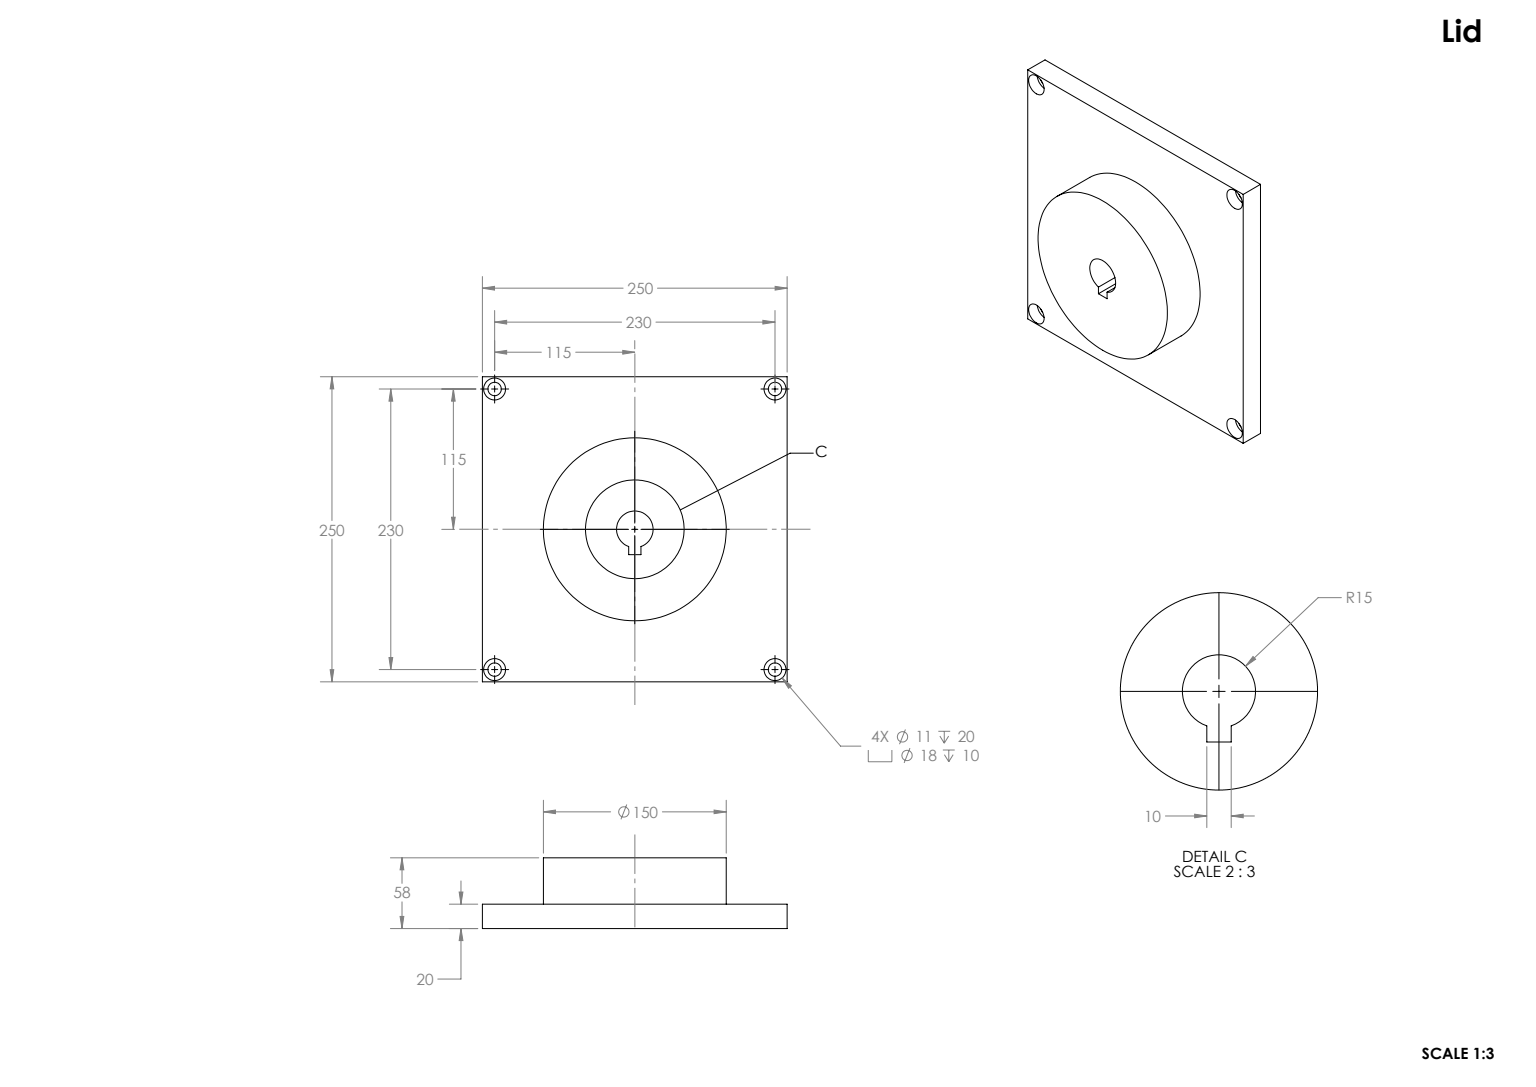
ISO-10303-21;
HEADER;
FILE_DESCRIPTION (('STEP AP214'),
    '1' );
FILE_NAME ('Lid.step',
    '2026-10-28T15:55:38',
    ( '' ),
    ( '' ),
    'SwSTEP 2.0',
    'SolidWorks 2025',
    '' );
FILE_SCHEMA (( 'AUTOMOTIVE_DESIGN' ));
ENDSEC;

DATA;
#6=AXIS2_PLACEMENT_3D ( 'NONE', #6964, #1191, #3754 ) ;
#14=VERTEX_POINT ( 'NONE', #1674 ) ;
#22=DIRECTION ( 'NONE',  ( -0.000000000000000000, -0.000000000000000000, 1.000000000000000000 ) ) ;
#33=ADVANCED_FACE ( 'NONE', ( #7283, #3451 ), #1624, .F. ) ;
#45=CARTESIAN_POINT ( 'NONE',  ( 0.000000000000000000, 0.000000000000000000, 57.99999999999999289 ) ) ;
#51=EDGE_CURVE ( 'NONE', #2241, #1087, #5313, .T. ) ;
#54=CARTESIAN_POINT ( 'NONE',  ( 115.0000000000000000, 114.9999999999999716, 10.00000000000000000 ) ) ;
#57=VERTEX_POINT ( 'NONE', #5409 ) ;
#69=VECTOR ( 'NONE', #3861, 1000.000000000000000 ) ;
#73=DIRECTION ( 'NONE',  ( -1.000000000000000000, -0.000000000000000000, -0.000000000000000000 ) ) ;
#77=APPLICATION_CONTEXT ( 'automotive_design' ) ;
#85=ORIENTED_EDGE ( 'NONE', *, *, #3477, .F. ) ;
#88=AXIS2_PLACEMENT_3D ( 'NONE', #5932, #1987, #3343 ) ;
#95=DIRECTION ( 'NONE',  ( -0.000000000000000000, -0.000000000000000000, 1.000000000000000000 ) ) ;
#99=ORIENTED_EDGE ( 'NONE', *, *, #619, .T. ) ;
#103=FACE_OUTER_BOUND ( 'NONE', #252, .T. ) ;
#107=CIRCLE ( 'NONE', #1347, 5.499999999999991118 ) ;
#117=FACE_OUTER_BOUND ( 'NONE', #1113, .T. ) ;
#119=AXIS2_PLACEMENT_3D ( 'NONE', #3115, #5695, #7738 ) ;
#121=DIRECTION ( 'NONE',  ( -0.000000000000000000, -0.000000000000000000, 1.000000000000000000 ) ) ;
#125=ORIENTED_EDGE ( 'NONE', *, *, #5217, .T. ) ;
#126=PLANE ( 'NONE',  #6282 ) ;
#129=ORIENTED_EDGE ( 'NONE', *, *, #3717, .T. ) ;
#133=CARTESIAN_POINT ( 'NONE',  ( 14.14213562373095279, -5.000000000000000000, 0.000000000000000000 ) ) ;
#134=ADVANCED_FACE ( 'NONE', ( #2899 ), #7943, .F. ) ;
#140=AXIS2_PLACEMENT_3D ( 'NONE', #6010, #7299, #1005 ) ;
#144=CARTESIAN_POINT ( 'NONE',  ( -109.5000000000000000, -114.9999999999999858, 20.00000000000000000 ) ) ;
#153=VERTEX_POINT ( 'NONE', #5449 ) ;
#156=DIRECTION ( 'NONE',  ( 1.000000000000000000, 0.000000000000000000, 0.000000000000000000 ) ) ;
#166=CARTESIAN_POINT ( 'NONE',  ( 124.9999999999997442, -125.0000000000000000, 20.00000000000000000 ) ) ;
#189=EDGE_CURVE ( 'NONE', #2853, #6262, #8132, .T. ) ;
#197=CARTESIAN_POINT ( 'NONE',  ( 115.0000000000000000, 114.9999999999999716, 10.00000000000000000 ) ) ;
#218=ORIENTED_EDGE ( 'NONE', *, *, #2588, .F. ) ;
#235=DIRECTION ( 'NONE',  ( 1.000000000000000000, 0.000000000000000000, 0.000000000000000000 ) ) ;
#252=EDGE_LOOP ( 'NONE', ( #5794, #5594, #8327, #2636 ) ) ;
#253=VECTOR ( 'NONE', #4816, 1000.000000000000000 ) ;
#258=ADVANCED_FACE ( 'NONE', ( #117 ), #4551, .F. ) ;
#259=DIRECTION ( 'NONE',  ( 9.992007221626408864E-16, 1.000000000000000000, 0.000000000000000000 ) ) ;
#268=VERTEX_POINT ( 'NONE', #3361 ) ;
#273=ORIENTED_EDGE ( 'NONE', *, *, #5206, .F. ) ;
#274=DIRECTION ( 'NONE',  ( 0.000000000000000000, -0.000000000000000000, -1.000000000000000000 ) ) ;
#283=ADVANCED_FACE ( 'NONE', ( #3284, #3966, #689, #5244, #1367, #6459 ), #5952, .F. ) ;
#284=EDGE_CURVE ( 'NONE', #5879, #3698, #7868, .T. ) ;
#290=ORIENTED_EDGE ( 'NONE', *, *, #7886, .F. ) ;
#293=VERTEX_POINT ( 'NONE', #814 ) ;
#299=APPLICATION_CONTEXT ( 'automotive_design' ) ;
#312=EDGE_LOOP ( 'NONE', ( #3163, #5141 ) ) ;
#317=CARTESIAN_POINT ( 'NONE',  ( 125.0000000000000000, 125.0000000000000000, 0.000000000000000000 ) ) ;
#322=DIRECTION ( 'NONE',  ( -0.000000000000000000, -0.000000000000000000, -1.000000000000000000 ) ) ;
#351=VERTEX_POINT ( 'NONE', #1784 ) ;
#353=DIRECTION ( 'NONE',  ( 1.000000000000000000, 0.000000000000000000, 0.000000000000000000 ) ) ;
#361=DIRECTION ( 'NONE',  ( 1.000000000000000000, 0.000000000000000000, 0.000000000000000000 ) ) ;
#365=ORIENTED_EDGE ( 'NONE', *, *, #7229, .F. ) ;
#369=CARTESIAN_POINT ( 'NONE',  ( 20.76917701662883076, -5.000000000000000000, 0.000000000000000000 ) ) ;
#372=VERTEX_POINT ( 'NONE', #4240 ) ;
#379=ORIENTED_EDGE ( 'NONE', *, *, #688, .F. ) ;
#426=VERTEX_POINT ( 'NONE', #6449 ) ;
#432=CARTESIAN_POINT ( 'NONE',  ( 124.0000000000000000, 114.9999999999999716, 10.00000000000000000 ) ) ;
#438=ORIENTED_EDGE ( 'NONE', *, *, #5217, .F. ) ;
#442=LINE ( 'NONE', #6912, #6022 ) ;
#449=DIRECTION ( 'NONE',  ( -1.000000000000000000, 0.000000000000000000, -0.000000000000000000 ) ) ;
#462=EDGE_CURVE ( 'NONE', #1143, #501, #4654, .T. ) ;
#464=( GEOMETRIC_REPRESENTATION_CONTEXT ( 3 ) GLOBAL_UNCERTAINTY_ASSIGNED_CONTEXT ( ( #4359 ) ) GLOBAL_UNIT_ASSIGNED_CONTEXT ( ( #3691, #7766, #3944 ) ) REPRESENTATION_CONTEXT ( 'NONE', 'WORKASPACE' ) );
#482=CIRCLE ( 'NONE', #7640, 8.999999999999994671 ) ;
#498=DIRECTION ( 'NONE',  ( -1.000000000000000000, -0.000000000000000000, -0.000000000000000000 ) ) ;
#501=VERTEX_POINT ( 'NONE', #1652 ) ;
#504=AXIS2_PLACEMENT_3D ( 'NONE', #7381, #3470, #967 ) ;
#514=ORIENTED_EDGE ( 'NONE', *, *, #1744, .T. ) ;
#521=ORIENTED_EDGE ( 'NONE', *, *, #5929, .F. ) ;
#542=ORIENTED_EDGE ( 'NONE', *, *, #6069, .T. ) ;
#561=EDGE_LOOP ( 'NONE', ( #1225, #8285, #5177, #3711 ) ) ;
#571=EDGE_LOOP ( 'NONE', ( #8103, #3538 ) ) ;
#572=CARTESIAN_POINT ( 'NONE',  ( 0.000000000000000000, 0.000000000000000000, 57.99999999999999289 ) ) ;
#574=CARTESIAN_POINT ( 'NONE',  ( -105.9999999999999858, -114.9999999999999858, 20.00000000000000000 ) ) ;
#577=AXIS2_PLACEMENT_3D ( 'NONE', #4578, #1221, #3947 ) ;
#586=LINE ( 'NONE', #6396, #3892 ) ;
#601=ORIENTED_EDGE ( 'NONE', *, *, #7179, .F. ) ;
#616=DIRECTION ( 'NONE',  ( -0.000000000000000000, -0.000000000000000000, 1.000000000000000000 ) ) ;
#619=EDGE_CURVE ( 'NONE', #372, #3698, #5183, .T. ) ;
#625=EDGE_LOOP ( 'NONE', ( #5499, #7571, #8014, #125 ) ) ;
#627=AXIS2_PLACEMENT_3D ( 'NONE', #6959, #2577, #1183 ) ;
#634=ORIENTED_EDGE ( 'NONE', *, *, #7886, .T. ) ;
#653=VERTEX_POINT ( 'NONE', #4478 ) ;
#655=CYLINDRICAL_SURFACE ( 'NONE', #1454, 75.00000000000001421 ) ;
#664=EDGE_CURVE ( 'NONE', #8205, #351, #3409, .T. ) ;
#667=ORIENTED_EDGE ( 'NONE', *, *, #3851, .F. ) ;
#669=CARTESIAN_POINT ( 'NONE',  ( 120.5000000000000000, 114.9999999999999716, 10.00000000000000000 ) ) ;
#685=VECTOR ( 'NONE', #498, 1000.000000000000000 ) ;
#686=CARTESIAN_POINT ( 'NONE',  ( -120.4999999999999858, -114.9999999999999858, 0.000000000000000000 ) ) ;
#688=EDGE_CURVE ( 'NONE', #7860, #57, #8154, .T. ) ;
#689=FACE_BOUND ( 'NONE', #7167, .T. ) ;
#716=CARTESIAN_POINT ( 'NONE',  ( 106.0000000000000142, -114.9999999999999716, 20.00000000000000000 ) ) ;
#719=VECTOR ( 'NONE', #8002, 1000.000000000000000 ) ;
#725=ADVANCED_FACE ( 'NONE', ( #4875 ), #7426, .F. ) ;
#732=LINE ( 'NONE', #8263, #8074 ) ;
#758=VERTEX_POINT ( 'NONE', #317 ) ;
#759=DIRECTION ( 'NONE',  ( -0.000000000000000000, -0.000000000000000000, 1.000000000000000000 ) ) ;
#768=DIRECTION ( 'NONE',  ( 1.000000000000000000, 0.000000000000000000, 0.000000000000000000 ) ) ;
#771=CARTESIAN_POINT ( 'NONE',  ( 75.00000000000001421, 9.184850993605150311E-15, 57.99999999999999289 ) ) ;
#780=CIRCLE ( 'NONE', #5493, 5.499999999999991118 ) ;
#790=VECTOR ( 'NONE', #7088, 1000.000000000000000 ) ;
#794=DIRECTION ( 'NONE',  ( -0.000000000000000000, -0.000000000000000000, 1.000000000000000000 ) ) ;
#799=AXIS2_PLACEMENT_3D ( 'NONE', #2892, #1645, #6922 ) ;
#809=ORIENTED_EDGE ( 'NONE', *, *, #1189, .T. ) ;
#814=CARTESIAN_POINT ( 'NONE',  ( 106.0000000000000142, 114.9999999999999716, 20.00000000000000000 ) ) ;
#818=DIRECTION ( 'NONE',  ( 1.000000000000000000, -9.992007221626408864E-16, 0.000000000000000000 ) ) ;
#826=MANIFOLD_SOLID_BREP ( 'CBORE for M10 SHCS1', #2352 ) ;
#837=EDGE_LOOP ( 'NONE', ( #1271, #3506, #2194, #809 ) ) ;
#844=CARTESIAN_POINT ( 'NONE',  ( -114.9999999999999716, 114.9999999999999858, 0.000000000000000000 ) ) ;
#853=CARTESIAN_POINT ( 'NONE',  ( 115.0000000000000000, -114.9999999999999716, 10.00000000000000000 ) ) ;
#873=AXIS2_PLACEMENT_3D ( 'NONE', #2320, #8006, #5392 ) ;
#886=DIRECTION ( 'NONE',  ( -0.000000000000000000, -0.000000000000000000, 1.000000000000000000 ) ) ;
#891=ADVANCED_BREP_SHAPE_REPRESENTATION ( '', ( #826, #1299 ), #3387 ) ;
#893=FACE_BOUND ( 'NONE', #1076, .T. ) ;
#898=LINE ( 'NONE', #5411, #1902 ) ;
#905=CARTESIAN_POINT ( 'NONE',  ( 0.000000000000000000, -5.000000000000000000, 57.99999999999999289 ) ) ;
#919=DIRECTION ( 'NONE',  ( -0.000000000000000000, -0.000000000000000000, 1.000000000000000000 ) ) ;
#924=ORIENTED_EDGE ( 'NONE', *, *, #2528, .T. ) ;
#927=AXIS2_PLACEMENT_3D ( 'NONE', #5655, #7690, #1908 ) ;
#929=VERTEX_POINT ( 'NONE', #6649 ) ;
#964=CARTESIAN_POINT ( 'NONE',  ( 115.0000000000000000, -114.9999999999999716, 0.000000000000000000 ) ) ;
#967=DIRECTION ( 'NONE',  ( 1.000000000000000000, 0.000000000000000000, 0.000000000000000000 ) ) ;
#971=FACE_OUTER_BOUND ( 'NONE', #1682, .T. ) ;
#979=DIRECTION ( 'NONE',  ( 1.000000000000000000, 0.000000000000000000, 0.000000000000000000 ) ) ;
#989=DIRECTION ( 'NONE',  ( -1.000000000000000000, 0.000000000000000000, -0.000000000000000000 ) ) ;
#992=CARTESIAN_POINT ( 'NONE',  ( -124.0000000000000000, -114.9999999999999858, 20.00000000000000000 ) ) ;
#995=LINE ( 'NONE', #2149, #5893 ) ;
#1005=DIRECTION ( 'NONE',  ( 1.000000000000000000, 0.000000000000000000, 0.000000000000000000 ) ) ;
#1009=DIRECTION ( 'NONE',  ( -0.000000000000000000, -0.000000000000000000, 1.000000000000000000 ) ) ;
#1014=DIRECTION ( 'NONE',  ( -9.992007221626408864E-16, -1.000000000000000000, -0.000000000000000000 ) ) ;
#1041=ORIENTED_EDGE ( 'NONE', *, *, #7075, .T. ) ;
#1047=AXIS2_PLACEMENT_3D ( 'NONE', #6210, #2387, #6762 ) ;
#1053=CARTESIAN_POINT ( 'NONE',  ( -125.0000000000000000, 125.0000000000000000, 20.00000000000000000 ) ) ;
#1065=CIRCLE ( 'NONE', #799, 8.999999999999994671 ) ;
#1076=EDGE_LOOP ( 'NONE', ( #5400, #6032 ) ) ;
#1078=( NAMED_UNIT ( * ) PLANE_ANGLE_UNIT ( ) SI_UNIT ( $, .RADIAN. ) );
#1087=VERTEX_POINT ( 'NONE', #3806 ) ;
#1089=EDGE_CURVE ( 'NONE', #6262, #268, #5748, .T. ) ;
#1105=ORIENTED_EDGE ( 'NONE', *, *, #2915, .T. ) ;
#1113=EDGE_LOOP ( 'NONE', ( #6418, #4791, #1621, #1265 ) ) ;
#1121=CARTESIAN_POINT ( 'NONE',  ( -125.0000000000002558, -125.0000000000000000, 0.000000000000000000 ) ) ;
#1131=DIRECTION ( 'NONE',  ( 0.000000000000000000, 0.000000000000000000, 1.000000000000000000 ) ) ;
#1143=VERTEX_POINT ( 'NONE', #686 ) ;
#1145=ORIENTED_EDGE ( 'NONE', *, *, #664, .F. ) ;
#1158=CARTESIAN_POINT ( 'NONE',  ( 115.0000000000000000, 114.9999999999999716, 0.000000000000000000 ) ) ;
#1165=EDGE_LOOP ( 'NONE', ( #6743, #6397, #4823, #4757 ) ) ;
#1172=LINE ( 'NONE', #2644, #69 ) ;
#1175=ORIENTED_EDGE ( 'NONE', *, *, #6340, .F. ) ;
#1183=DIRECTION ( 'NONE',  ( 1.000000000000000000, 0.000000000000000000, 0.000000000000000000 ) ) ;
#1187=PRODUCT_CONTEXT ( 'NONE', #77, 'mechanical' ) ;
#1189=EDGE_CURVE ( 'NONE', #5618, #268, #5155, .T. ) ;
#1191=DIRECTION ( 'NONE',  ( 0.000000000000000000, 0.000000000000000000, 1.000000000000000000 ) ) ;
#1192=VECTOR ( 'NONE', #2719, 1000.000000000000000 ) ;
#1199=VERTEX_POINT ( 'NONE', #2217 ) ;
#1200=CIRCLE ( 'NONE', #6849, 5.499999999999991118 ) ;
#1202=DIRECTION ( 'NONE',  ( 1.000000000000000000, 0.000000000000000000, 0.000000000000000000 ) ) ;
#1207=VERTEX_POINT ( 'NONE', #7349 ) ;
#1208=EDGE_CURVE ( 'NONE', #5352, #293, #1483, .T. ) ;
#1221=DIRECTION ( 'NONE',  ( -1.000000000000000000, 9.992007221626408864E-16, 0.000000000000000000 ) ) ;
#1225=ORIENTED_EDGE ( 'NONE', *, *, #1208, .F. ) ;
#1263=ORIENTED_EDGE ( 'NONE', *, *, #2767, .T. ) ;
#1265=ORIENTED_EDGE ( 'NONE', *, *, #1711, .T. ) ;
#1271=ORIENTED_EDGE ( 'NONE', *, *, #1089, .F. ) ;
#1294=VERTEX_POINT ( 'NONE', #5614 ) ;
#1296=CARTESIAN_POINT ( 'NONE',  ( -114.9999999999999858, -114.9999999999999858, 10.00000000000000000 ) ) ;
#1299=AXIS2_PLACEMENT_3D ( 'NONE', #5884, #1507, #5927 ) ;
#1300=ORIENTED_EDGE ( 'NONE', *, *, #2228, .F. ) ;
#1308=VECTOR ( 'NONE', #4861, 1000.000000000000000 ) ;
#1340=LINE ( 'NONE', #3907, #3449 ) ;
#1347=AXIS2_PLACEMENT_3D ( 'NONE', #2247, #2924, #1634 ) ;
#1349=EDGE_LOOP ( 'NONE', ( #1695, #7646 ) ) ;
#1358=LINE ( 'NONE', #6493, #7675 ) ;
#1362=ADVANCED_FACE ( 'NONE', ( #1991 ), #4621, .F. ) ;
#1366=ORIENTED_EDGE ( 'NONE', *, *, #7946, .F. ) ;
#1367=FACE_BOUND ( 'NONE', #3037, .T. ) ;
#1368=CARTESIAN_POINT ( 'NONE',  ( 124.0000000000000000, 114.9999999999999716, 20.00000000000000000 ) ) ;
#1372=ORIENTED_EDGE ( 'NONE', *, *, #2788, .F. ) ;
#1381=DIRECTION ( 'NONE',  ( -0.000000000000000000, -0.000000000000000000, 1.000000000000000000 ) ) ;
#1385=ORIENTED_EDGE ( 'NONE', *, *, #6069, .F. ) ;
#1417=AXIS2_PLACEMENT_3D ( 'NONE', #7031, #4519, #5124 ) ;
#1431=ORIENTED_EDGE ( 'NONE', *, *, #2734, .T. ) ;
#1435=VECTOR ( 'NONE', #259, 1000.000000000000000 ) ;
#1444=ORIENTED_EDGE ( 'NONE', *, *, #3717, .F. ) ;
#1447=DIRECTION ( 'NONE',  ( -0.000000000000000000, -0.000000000000000000, 1.000000000000000000 ) ) ;
#1450=EDGE_CURVE ( 'NONE', #6338, #1207, #1511, .T. ) ;
#1453=FACE_BOUND ( 'NONE', #6015, .T. ) ;
#1454=AXIS2_PLACEMENT_3D ( 'NONE', #572, #1894, #6985 ) ;
#1471=AXIS2_PLACEMENT_3D ( 'NONE', #3560, #7559, #361 ) ;
#1477=LINE ( 'NONE', #7862, #1605 ) ;
#1483=LINE ( 'NONE', #6755, #2989 ) ;
#1487=PRODUCT_DEFINITION_SHAPE ( 'NONE', 'NONE',  #1686 ) ;
#1495=FACE_BOUND ( 'NONE', #2408, .T. ) ;
#1503=CARTESIAN_POINT ( 'NONE',  ( -109.5000000000000000, -114.9999999999999858, 10.00000000000000000 ) ) ;
#1505=DIRECTION ( 'NONE',  ( -1.000000000000000000, 0.000000000000000000, -0.000000000000000000 ) ) ;
#1507=DIRECTION ( 'NONE',  ( 0.000000000000000000, 0.000000000000000000, 1.000000000000000000 ) ) ;
#1511=LINE ( 'NONE', #7201, #4061 ) ;
#1515=LINE ( 'NONE', #7334, #5232 ) ;
#1519=AXIS2_PLACEMENT_3D ( 'NONE', #197, #2821, #156 ) ;
#1533=EDGE_CURVE ( 'NONE', #1199, #153, #4022, .T. ) ;
#1535=FACE_OUTER_BOUND ( 'NONE', #3964, .T. ) ;
#1538=ORIENTED_EDGE ( 'NONE', *, *, #5058, .F. ) ;
#1548=ORIENTED_EDGE ( 'NONE', *, *, #3525, .T. ) ;
#1552=ORIENTED_EDGE ( 'NONE', *, *, #1450, .T. ) ;
#1557=DIRECTION ( 'NONE',  ( 1.000000000000000000, 0.000000000000000000, 0.000000000000000000 ) ) ;
#1566=VERTEX_POINT ( 'NONE', #6176 ) ;
#1567=CARTESIAN_POINT ( 'NONE',  ( 125.0000000000000000, 125.0000000000000000, 20.00000000000000000 ) ) ;
#1568=DIRECTION ( 'NONE',  ( -0.000000000000000000, -0.000000000000000000, 1.000000000000000000 ) ) ;
#1605=VECTOR ( 'NONE', #2094, 1000.000000000000000 ) ;
#1615=CARTESIAN_POINT ( 'NONE',  ( 120.5000000000000000, 114.9999999999999716, 20.00000000000000000 ) ) ;
#1620=CIRCLE ( 'NONE', #7960, 75.00000000000001421 ) ;
#1621=ORIENTED_EDGE ( 'NONE', *, *, #7009, .T. ) ;
#1624=PLANE ( 'NONE',  #2738 ) ;
#1633=ORIENTED_EDGE ( 'NONE', *, *, #3223, .T. ) ;
#1634=DIRECTION ( 'NONE',  ( 1.000000000000000000, 0.000000000000000000, 0.000000000000000000 ) ) ;
#1636=EDGE_CURVE ( 'NONE', #3543, #5352, #2216, .T. ) ;
#1644=ORIENTED_EDGE ( 'NONE', *, *, #5930, .T. ) ;
#1645=DIRECTION ( 'NONE',  ( -0.000000000000000000, -0.000000000000000000, 1.000000000000000000 ) ) ;
#1652=CARTESIAN_POINT ( 'NONE',  ( -120.4999999999999858, -114.9999999999999858, 10.00000000000000000 ) ) ;
#1662=VERTEX_POINT ( 'NONE', #5987 ) ;
#1673=DIRECTION ( 'NONE',  ( 1.000000000000000000, 0.000000000000000000, 0.000000000000000000 ) ) ;
#1674=CARTESIAN_POINT ( 'NONE',  ( 120.5000000000000000, -114.9999999999999716, 0.000000000000000000 ) ) ;
#1682=EDGE_LOOP ( 'NONE', ( #8203, #4102, #5975, #2895 ) ) ;
#1686=PRODUCT_DEFINITION ( 'UNKNOWN', '', #2343, #7430 ) ;
#1695=ORIENTED_EDGE ( 'NONE', *, *, #189, .T. ) ;
#1698=EDGE_CURVE ( 'NONE', #3530, #2214, #6790, .T. ) ;
#1700=ADVANCED_FACE ( 'NONE', ( #6744 ), #8096, .F. ) ;
#1703=CIRCLE ( 'NONE', #4107, 9.000000000000007105 ) ;
#1708=SHAPE_REPRESENTATION ( 'Lid', ( #1299 ), #3387 ) ;
#1711=EDGE_CURVE ( 'NONE', #929, #501, #3521, .T. ) ;
#1721=AXIS2_PLACEMENT_3D ( 'NONE', #7158, #95, #6475 ) ;
#1727=AXIS2_PLACEMENT_3D ( 'NONE', #4123, #7941, #7907 ) ;
#1740=CARTESIAN_POINT ( 'NONE',  ( -114.9999999999999716, 114.9999999999999858, 10.00000000000000000 ) ) ;
#1744=EDGE_CURVE ( 'NONE', #3799, #4692, #4066, .T. ) ;
#1750=VECTOR ( 'NONE', #7803, 1000.000000000000000 ) ;
#1754=EDGE_LOOP ( 'NONE', ( #5016, #1300, #6482, #2342 ) ) ;
#1762=ORIENTED_EDGE ( 'NONE', *, *, #2056, .T. ) ;
#1779=SHAPE_DEFINITION_REPRESENTATION ( #1487, #1708 ) ;
#1784=CARTESIAN_POINT ( 'NONE',  ( 14.14213562373095279, -5.000000000000000000, 0.000000000000000000 ) ) ;
#1791=ORIENTED_EDGE ( 'NONE', *, *, #1450, .F. ) ;
#1817=EDGE_CURVE ( 'NONE', #6862, #1662, #6546, .T. ) ;
#1822=DIRECTION ( 'NONE',  ( -0.000000000000000000, -0.000000000000000000, 1.000000000000000000 ) ) ;
#1825=CARTESIAN_POINT ( 'NONE',  ( 20.76917701662883076, -5.000000000000000000, 57.99999999999999289 ) ) ;
#1842=ORIENTED_EDGE ( 'NONE', *, *, #1698, .T. ) ;
#1848=AXIS2_PLACEMENT_3D ( 'NONE', #45, #7313, #3973 ) ;
#1849=CIRCLE ( 'NONE', #6559, 75.00000000000001421 ) ;
#1861=CARTESIAN_POINT ( 'NONE',  ( -114.9999999999999716, 114.9999999999999858, 20.00000000000000000 ) ) ;
#1874=EDGE_LOOP ( 'NONE', ( #1791, #8170, #4052, #6913 ) ) ;
#1887=CIRCLE ( 'NONE', #1471, 8.999999999999994671 ) ;
#1889=VERTEX_POINT ( 'NONE', #2953 ) ;
#1892=AXIS2_PLACEMENT_3D ( 'NONE', #4105, #7499, #5471 ) ;
#1894=DIRECTION ( 'NONE',  ( -0.000000000000000000, -0.000000000000000000, -1.000000000000000000 ) ) ;
#1898=DIRECTION ( 'NONE',  ( -0.000000000000000000, -0.000000000000000000, 1.000000000000000000 ) ) ;
#1902=VECTOR ( 'NONE', #2179, 1000.000000000000000 ) ;
#1903=CARTESIAN_POINT ( 'NONE',  ( -114.9999999999999858, -114.9999999999999858, 10.00000000000000000 ) ) ;
#1908=DIRECTION ( 'NONE',  ( 1.000000000000000000, 0.000000000000000000, 0.000000000000000000 ) ) ;
#1909=DIRECTION ( 'NONE',  ( 1.000000000000000000, 0.000000000000000000, 0.000000000000000000 ) ) ;
#1945=PLANE ( 'NONE',  #88 ) ;
#1958=AXIS2_PLACEMENT_3D ( 'NONE', #7833, #3321, #2667 ) ;
#1966=EDGE_CURVE ( 'NONE', #2083, #8025, #7305, .T. ) ;
#1987=DIRECTION ( 'NONE',  ( -1.000000000000000000, 0.000000000000000000, -0.000000000000000000 ) ) ;
#1991=FACE_OUTER_BOUND ( 'NONE', #5640, .T. ) ;
#2007=AXIS2_PLACEMENT_3D ( 'NONE', #7496, #7627, #6901 ) ;
#2025=FACE_OUTER_BOUND ( 'NONE', #7078, .T. ) ;
#2036=AXIS2_PLACEMENT_3D ( 'NONE', #964, #6773, #2282 ) ;
#2038=FACE_OUTER_BOUND ( 'NONE', #3344, .T. ) ;
#2041=VERTEX_POINT ( 'NONE', #6787 ) ;
#2042=FACE_OUTER_BOUND ( 'NONE', #6018, .T. ) ;
#2045=EDGE_LOOP ( 'NONE', ( #1633, #379, #4234, #5708 ) ) ;
#2054=ORIENTED_EDGE ( 'NONE', *, *, #2757, .F. ) ;
#2056=EDGE_CURVE ( 'NONE', #8025, #1889, #4282, .T. ) ;
#2082=FACE_OUTER_BOUND ( 'NONE', #561, .T. ) ;
#2083=VERTEX_POINT ( 'NONE', #1567 ) ;
#2094=DIRECTION ( 'NONE',  ( -0.000000000000000000, -0.000000000000000000, 1.000000000000000000 ) ) ;
#2103=CARTESIAN_POINT ( 'NONE',  ( -125.0000000000002558, -125.0000000000000000, 20.00000000000000000 ) ) ;
#2111=STYLED_ITEM('',(#8386),#826);
#2114=LINE ( 'NONE', #4656, #1435 ) ;
#2120=DIRECTION ( 'NONE',  ( -0.000000000000000000, -0.000000000000000000, 1.000000000000000000 ) ) ;
#2149=CARTESIAN_POINT ( 'NONE',  ( 120.5000000000000000, -114.9999999999999716, 20.00000000000000000 ) ) ;
#2174=EDGE_CURVE ( 'NONE', #4652, #293, #4596, .T. ) ;
#2179=DIRECTION ( 'NONE',  ( 1.000000000000000000, 0.000000000000000000, 0.000000000000000000 ) ) ;
#2187=DIRECTION ( 'NONE',  ( -0.000000000000000000, -0.000000000000000000, -1.000000000000000000 ) ) ;
#2194=ORIENTED_EDGE ( 'NONE', *, *, #6340, .T. ) ;
#2198=DIRECTION ( 'NONE',  ( 1.000000000000000000, 0.000000000000000000, 0.000000000000000000 ) ) ;
#2211=EDGE_LOOP ( 'NONE', ( #6715, #5144 ) ) ;
#2214=VERTEX_POINT ( 'NONE', #1825 ) ;
#2216=CIRCLE ( 'NONE', #5703, 8.999999999999994671 ) ;
#2217=CARTESIAN_POINT ( 'NONE',  ( -105.9999999999999858, 114.9999999999999858, 10.00000000000000000 ) ) ;
#2225=CARTESIAN_POINT ( 'NONE',  ( -125.0000000000000000, 125.0000000000000000, 0.000000000000000000 ) ) ;
#2228=EDGE_CURVE ( 'NONE', #5826, #6862, #6209, .T. ) ;
#2231=EDGE_LOOP ( 'NONE', ( #6208, #6016, #4285, #1175 ) ) ;
#2241=VERTEX_POINT ( 'NONE', #716 ) ;
#2247=CARTESIAN_POINT ( 'NONE',  ( 115.0000000000000000, -114.9999999999999716, 10.00000000000000000 ) ) ;
#2271=LINE ( 'NONE', #1121, #1308 ) ;
#2274=DIRECTION ( 'NONE',  ( 1.000000000000000000, 0.000000000000000000, 0.000000000000000000 ) ) ;
#2282=DIRECTION ( 'NONE',  ( 1.000000000000000000, 0.000000000000000000, 0.000000000000000000 ) ) ;
#2288=CARTESIAN_POINT ( 'NONE',  ( 120.5000000000000000, -114.9999999999999716, 10.00000000000000000 ) ) ;
#2302=AXIS2_PLACEMENT_3D ( 'NONE', #6884, #6796, #6154 ) ;
#2307=DIRECTION ( 'NONE',  ( 0.000000000000000000, 0.000000000000000000, -1.000000000000000000 ) ) ;
#2309=EDGE_LOOP ( 'NONE', ( #6537, #7695 ) ) ;
#2320=CARTESIAN_POINT ( 'NONE',  ( -114.9999999999999716, 114.9999999999999858, 20.00000000000000000 ) ) ;
#2324=CIRCLE ( 'NONE', #140, 5.499999999999991118 ) ;
#2325=CARTESIAN_POINT ( 'NONE',  ( 0.000000000000000000, 0.000000000000000000, 0.000000000000000000 ) ) ;
#2329=ORIENTED_EDGE ( 'NONE', *, *, #7065, .F. ) ;
#2333=ORIENTED_EDGE ( 'NONE', *, *, #1966, .T. ) ;
#2342=ORIENTED_EDGE ( 'NONE', *, *, #7806, .T. ) ;
#2343=PRODUCT_DEFINITION_FORMATION_WITH_SPECIFIED_SOURCE ( 'ANY', '', #6606, .NOT_KNOWN. ) ;
#2352=CLOSED_SHELL ( 'NONE', ( #2529, #8144, #3128, #5215, #2963, #5368, #2826, #3278, #4237, #5306, #134, #4458, #1362, #3668, #283, #8202, #4201, #1700, #8082, #2696, #5638, #258, #33, #7694, #6228, #5403, #8167, #4433, #3480, #5686, #725, #4774, #2725 ) ) ;
#2353=ORIENTED_EDGE ( 'NONE', *, *, #7980, .T. ) ;
#2361=EDGE_LOOP ( 'NONE', ( #8298, #1263, #5982, #365 ) ) ;
#2380=CYLINDRICAL_SURFACE ( 'NONE', #2302, 5.499999999999991118 ) ;
#2387=DIRECTION ( 'NONE',  ( 0.000000000000000000, 1.000000000000000000, 0.000000000000000000 ) ) ;
#2408=EDGE_LOOP ( 'NONE', ( #438, #7740 ) ) ;
#2429=EDGE_CURVE ( 'NONE', #501, #929, #2324, .T. ) ;
#2444=CARTESIAN_POINT ( 'NONE',  ( 20.76917701662883076, 0.000000000000000000, 0.000000000000000000 ) ) ;
#2454=UNCERTAINTY_MEASURE_WITH_UNIT (LENGTH_MEASURE( 1.000000000000000082E-05 ), #5550, 'distance_accuracy_value', 'NONE');
#2509=CARTESIAN_POINT ( 'NONE',  ( -75.00000000000001421, 0.000000000000000000, 20.00000000000000000 ) ) ;
#2514=DIRECTION ( 'NONE',  ( -0.000000000000000000, -0.000000000000000000, 1.000000000000000000 ) ) ;
#2522=CARTESIAN_POINT ( 'NONE',  ( -114.9999999999999858, -114.9999999999999858, 20.00000000000000000 ) ) ;
#2524=DIRECTION ( 'NONE',  ( -0.000000000000000000, -0.000000000000000000, 1.000000000000000000 ) ) ;
#2528=EDGE_CURVE ( 'NONE', #4692, #3799, #2540, .T. ) ;
#2529=ADVANCED_FACE ( 'NONE', ( #4225 ), #3601, .F. ) ;
#2533=ORIENTED_EDGE ( 'NONE', *, *, #4785, .F. ) ;
#2537=DIRECTION ( 'NONE',  ( 1.000000000000000000, 0.000000000000000000, 0.000000000000000000 ) ) ;
#2540=CIRCLE ( 'NONE', #7118, 9.000000000000007105 ) ;
#2545=AXIS2_PLACEMENT_3D ( 'NONE', #844, #759, #5351 ) ;
#2555=ORIENTED_EDGE ( 'NONE', *, *, #2912, .F. ) ;
#2577=DIRECTION ( 'NONE',  ( -0.000000000000000000, -0.000000000000000000, 1.000000000000000000 ) ) ;
#2584=CARTESIAN_POINT ( 'NONE',  ( -125.0000000000002558, -125.0000000000000000, 0.000000000000000000 ) ) ;
#2588=EDGE_CURVE ( 'NONE', #8205, #7327, #442, .T. ) ;
#2618=FACE_OUTER_BOUND ( 'NONE', #625, .T. ) ;
#2626=ORIENTED_EDGE ( 'NONE', *, *, #8258, .F. ) ;
#2628=MECHANICAL_DESIGN_GEOMETRIC_PRESENTATION_REPRESENTATION('',(#2111),#464);
#2631=CARTESIAN_POINT ( 'NONE',  ( -109.4999999999999858, 114.9999999999999858, 20.00000000000000000 ) ) ;
#2636=ORIENTED_EDGE ( 'NONE', *, *, #4631, .F. ) ;
#2637=FACE_BOUND ( 'NONE', #7473, .T. ) ;
#2641=FACE_OUTER_BOUND ( 'NONE', #6826, .T. ) ;
#2644=CARTESIAN_POINT ( 'NONE',  ( -125.0000000000002558, -125.0000000000000000, 20.00000000000000000 ) ) ;
#2645=AXIS2_PLACEMENT_3D ( 'NONE', #1861, #1822, #2537 ) ;
#2667=DIRECTION ( 'NONE',  ( 1.000000000000000000, 0.000000000000000000, -0.000000000000000000 ) ) ;
#2674=VERTEX_POINT ( 'NONE', #5084 ) ;
#2680=EDGE_LOOP ( 'NONE', ( #1548, #2626, #5631, #3946 ) ) ;
#2696=ADVANCED_FACE ( 'NONE', ( #2038 ), #1945, .T. ) ;
#2700=DIRECTION ( 'NONE',  ( 1.000000000000000000, 0.000000000000000000, 0.000000000000000000 ) ) ;
#2701=ORIENTED_EDGE ( 'NONE', *, *, #3345, .T. ) ;
#2719=DIRECTION ( 'NONE',  ( -0.000000000000000000, -0.000000000000000000, -1.000000000000000000 ) ) ;
#2725=ADVANCED_FACE ( 'NONE', ( #7808 ), #7199, .F. ) ;
#2734=EDGE_CURVE ( 'NONE', #1294, #7972, #4807, .T. ) ;
#2738=AXIS2_PLACEMENT_3D ( 'NONE', #1503, #2307, #989 ) ;
#2744=CARTESIAN_POINT ( 'NONE',  ( 20.76917701662883076, 5.000000000000000000, 0.000000000000000000 ) ) ;
#2748=EDGE_LOOP ( 'NONE', ( #129, #5296, #1145, #4036 ) ) ;
#2757=EDGE_CURVE ( 'NONE', #8025, #2041, #7241, .T. ) ;
#2767=EDGE_CURVE ( 'NONE', #4692, #7479, #1340, .T. ) ;
#2780=PLANE ( 'NONE',  #5358 ) ;
#2788=EDGE_CURVE ( 'NONE', #4729, #1566, #5129, .T. ) ;
#2800=DIRECTION ( 'NONE',  ( -0.000000000000000000, -0.000000000000000000, 1.000000000000000000 ) ) ;
#2812=EDGE_LOOP ( 'NONE', ( #667, #273, #7246, #5388 ) ) ;
#2821=DIRECTION ( 'NONE',  ( -0.000000000000000000, -0.000000000000000000, 1.000000000000000000 ) ) ;
#2822=EDGE_CURVE ( 'NONE', #14, #6508, #995, .T. ) ;
#2823=CARTESIAN_POINT ( 'NONE',  ( 109.5000000000000142, -114.9999999999999716, 0.000000000000000000 ) ) ;
#2826=ADVANCED_FACE ( 'NONE', ( #6650 ), #4060, .F. ) ;
#2840=CARTESIAN_POINT ( 'NONE',  ( -114.9999999999999858, -114.9999999999999858, 20.00000000000000000 ) ) ;
#2842=CARTESIAN_POINT ( 'NONE',  ( -105.9999999999999858, 114.9999999999999858, 20.00000000000000000 ) ) ;
#2845=CARTESIAN_POINT ( 'NONE',  ( 20.76917701662883076, 5.000000000000000000, 57.99999999999999289 ) ) ;
#2852=DIRECTION ( 'NONE',  ( -0.000000000000000000, -0.000000000000000000, 1.000000000000000000 ) ) ;
#2853=VERTEX_POINT ( 'NONE', #6768 ) ;
#2890=FACE_BOUND ( 'NONE', #8086, .T. ) ;
#2892=CARTESIAN_POINT ( 'NONE',  ( 115.0000000000000000, -114.9999999999999716, 10.00000000000000000 ) ) ;
#2895=ORIENTED_EDGE ( 'NONE', *, *, #2822, .F. ) ;
#2899=FACE_OUTER_BOUND ( 'NONE', #2680, .T. ) ;
#2909=PLANE ( 'NONE',  #1047 ) ;
#2912=EDGE_CURVE ( 'NONE', #1207, #153, #6699, .T. ) ;
#2915=EDGE_CURVE ( 'NONE', #1143, #426, #780, .T. ) ;
#2924=DIRECTION ( 'NONE',  ( -0.000000000000000000, -0.000000000000000000, 1.000000000000000000 ) ) ;
#2946=DIRECTION ( 'NONE',  ( -0.000000000000000000, -0.000000000000000000, 1.000000000000000000 ) ) ;
#2953=CARTESIAN_POINT ( 'NONE',  ( -125.0000000000002558, -125.0000000000000000, 20.00000000000000000 ) ) ;
#2954=EDGE_LOOP ( 'NONE', ( #1372, #2329, #4010, #542 ) ) ;
#2957=CYLINDRICAL_SURFACE ( 'NONE', #4804, 5.499999999999991118 ) ;
#2963=ADVANCED_FACE ( 'NONE', ( #3970 ), #7224, .F. ) ;
#2978=ORIENTED_EDGE ( 'NONE', *, *, #664, .T. ) ;
#2989=VECTOR ( 'NONE', #1568, 1000.000000000000000 ) ;
#2997=DIRECTION ( 'NONE',  ( -0.000000000000000000, -0.000000000000000000, 1.000000000000000000 ) ) ;
#3017=FACE_OUTER_BOUND ( 'NONE', #8250, .T. ) ;
#3019=ORIENTED_EDGE ( 'NONE', *, *, #5206, .T. ) ;
#3021=FACE_OUTER_BOUND ( 'NONE', #5891, .T. ) ;
#3033=CARTESIAN_POINT ( 'NONE',  ( 109.5000000000000142, 114.9999999999999716, 0.000000000000000000 ) ) ;
#3036=EDGE_CURVE ( 'NONE', #3698, #372, #7673, .T. ) ;
#3037=EDGE_LOOP ( 'NONE', ( #85, #2978, #5901, #521 ) ) ;
#3042=DIRECTION ( 'NONE',  ( -0.000000000000000000, -0.000000000000000000, 1.000000000000000000 ) ) ;
#3057=AXIS2_PLACEMENT_3D ( 'NONE', #7415, #4822, #4743 ) ;
#3060=EDGE_LOOP ( 'NONE', ( #1041, #1105 ) ) ;
#3062=ORIENTED_EDGE ( 'NONE', *, *, #5281, .F. ) ;
#3076=VECTOR ( 'NONE', #2120, 1000.000000000000000 ) ;
#3085=CIRCLE ( 'NONE', #1892, 5.499999999999991118 ) ;
#3093=CYLINDRICAL_SURFACE ( 'NONE', #4287, 9.000000000000007105 ) ;
#3098=VECTOR ( 'NONE', #6758, 1000.000000000000000 ) ;
#3099=LINE ( 'NONE', #5718, #4248 ) ;
#3115=CARTESIAN_POINT ( 'NONE',  ( 0.000000000000000000, 0.000000000000000000, 20.00000000000000000 ) ) ;
#3120=VERTEX_POINT ( 'NONE', #4067 ) ;
#3124=ORIENTED_EDGE ( 'NONE', *, *, #51, .T. ) ;
#3128=ADVANCED_FACE ( 'NONE', ( #103 ), #7378, .F. ) ;
#3136=VECTOR ( 'NONE', #2946, 1000.000000000000000 ) ;
#3163=ORIENTED_EDGE ( 'NONE', *, *, #1711, .F. ) ;
#3223=EDGE_CURVE ( 'NONE', #5090, #57, #1515, .T. ) ;
#3242=ORIENTED_EDGE ( 'NONE', *, *, #5058, .T. ) ;
#3259=DIRECTION ( 'NONE',  ( -0.000000000000000000, -0.000000000000000000, 1.000000000000000000 ) ) ;
#3278=ADVANCED_FACE ( 'NONE', ( #4911 ), #7548, .F. ) ;
#3284=FACE_BOUND ( 'NONE', #5189, .T. ) ;
#3310=CARTESIAN_POINT ( 'NONE',  ( 115.0000000000000000, -114.9999999999999716, 20.00000000000000000 ) ) ;
#3315=AXIS2_PLACEMENT_3D ( 'NONE', #3901, #8342, #5844 ) ;
#3316=AXIS2_PLACEMENT_3D ( 'NONE', #2840, #7368, #5337 ) ;
#3321=DIRECTION ( 'NONE',  ( 0.000000000000000000, 0.000000000000000000, 1.000000000000000000 ) ) ;
#3339=CARTESIAN_POINT ( 'NONE',  ( 0.000000000000000000, 5.000000000000000000, 0.000000000000000000 ) ) ;
#3343=DIRECTION ( 'NONE',  ( -0.000000000000000000, 0.000000000000000000, 1.000000000000000000 ) ) ;
#3344=EDGE_LOOP ( 'NONE', ( #3062, #290, #4509, #1842 ) ) ;
#3345=EDGE_CURVE ( 'NONE', #6862, #5826, #1849, .T. ) ;
#3352=CARTESIAN_POINT ( 'NONE',  ( 115.0000000000000000, 114.9999999999999716, 20.00000000000000000 ) ) ;
#3361=CARTESIAN_POINT ( 'NONE',  ( 109.5000000000000142, 114.9999999999999716, 10.00000000000000000 ) ) ;
#3363=AXIS2_PLACEMENT_3D ( 'NONE', #6240, #8238, #5740 ) ;
#3373=CARTESIAN_POINT ( 'NONE',  ( 0.000000000000000000, 0.000000000000000000, 0.000000000000000000 ) ) ;
#3387=( GEOMETRIC_REPRESENTATION_CONTEXT ( 3 ) GLOBAL_UNCERTAINTY_ASSIGNED_CONTEXT ( ( #2454 ) ) GLOBAL_UNIT_ASSIGNED_CONTEXT ( ( #5550, #1078, #4945 ) ) REPRESENTATION_CONTEXT ( 'NONE', 'WORKASPACE' ) );
#3391=DIRECTION ( 'NONE',  ( -0.000000000000000000, -0.000000000000000000, 1.000000000000000000 ) ) ;
#3392=ORIENTED_EDGE ( 'NONE', *, *, #6689, .T. ) ;
#3401=DIRECTION ( 'NONE',  ( 1.000000000000000000, 0.000000000000000000, 0.000000000000000000 ) ) ;
#3404=CARTESIAN_POINT ( 'NONE',  ( -109.4999999999999858, 114.9999999999999858, 10.00000000000000000 ) ) ;
#3409=CIRCLE ( 'NONE', #3546, 15.00000000000000178 ) ;
#3411=CARTESIAN_POINT ( 'NONE',  ( 124.9999999999997442, -125.0000000000000000, 20.00000000000000000 ) ) ;
#3415=EDGE_CURVE ( 'NONE', #7860, #2083, #2114, .T. ) ;
#3425=DIRECTION ( 'NONE',  ( -0.000000000000000000, -0.000000000000000000, 1.000000000000000000 ) ) ;
#3433=LINE ( 'NONE', #6017, #7819 ) ;
#3449=VECTOR ( 'NONE', #1381, 1000.000000000000000 ) ;
#3451=FACE_OUTER_BOUND ( 'NONE', #8292, .T. ) ;
#3457=DIRECTION ( 'NONE',  ( -0.000000000000000000, -0.000000000000000000, 1.000000000000000000 ) ) ;
#3470=DIRECTION ( 'NONE',  ( -0.000000000000000000, -0.000000000000000000, 1.000000000000000000 ) ) ;
#3476=DIRECTION ( 'NONE',  ( 0.000000000000000000, -1.000000000000000000, 0.000000000000000000 ) ) ;
#3477=EDGE_CURVE ( 'NONE', #8205, #5186, #7197, .T. ) ;
#3480=ADVANCED_FACE ( 'NONE', ( #4018, #4094 ), #4701, .F. ) ;
#3506=ORIENTED_EDGE ( 'NONE', *, *, #189, .F. ) ;
#3521=CIRCLE ( 'NONE', #3817, 5.499999999999991118 ) ;
#3525=EDGE_CURVE ( 'NONE', #2041, #5090, #2271, .T. ) ;
#3530=VERTEX_POINT ( 'NONE', #4818 ) ;
#3534=FACE_OUTER_BOUND ( 'NONE', #2045, .T. ) ;
#3538=ORIENTED_EDGE ( 'NONE', *, *, #8207, .T. ) ;
#3543=VERTEX_POINT ( 'NONE', #432 ) ;
#3546=AXIS2_PLACEMENT_3D ( 'NONE', #3373, #6725, #5581 ) ;
#3556=CARTESIAN_POINT ( 'NONE',  ( -114.9999999999999858, -114.9999999999999858, 10.00000000000000000 ) ) ;
#3560=CARTESIAN_POINT ( 'NONE',  ( -114.9999999999999716, 114.9999999999999858, 10.00000000000000000 ) ) ;
#3564=CIRCLE ( 'NONE', #8178, 9.000000000000007105 ) ;
#3600=AXIS2_PLACEMENT_3D ( 'NONE', #3310, #3391, #2700 ) ;
#3601=CYLINDRICAL_SURFACE ( 'NONE', #504, 8.999999999999994671 ) ;
#3604=CIRCLE ( 'NONE', #927, 8.999999999999994671 ) ;
#3617=DIRECTION ( 'NONE',  ( 1.000000000000000000, 0.000000000000000000, 0.000000000000000000 ) ) ;
#3625=AXIS2_PLACEMENT_3D ( 'NONE', #6875, #6236, #5609 ) ;
#3668=ADVANCED_FACE ( 'NONE', ( #1453, #2637, #1495, #4008, #6600, #1535 ), #126, .T. ) ;
#3691=( LENGTH_UNIT ( ) NAMED_UNIT ( * ) SI_UNIT ( .MILLI., .METRE. ) );
#3698=VERTEX_POINT ( 'NONE', #3404 ) ;
#3701=ORIENTED_EDGE ( 'NONE', *, *, #7946, .T. ) ;
#3704=ORIENTED_EDGE ( 'NONE', *, *, #7980, .F. ) ;
#3711=ORIENTED_EDGE ( 'NONE', *, *, #2174, .T. ) ;
#3717=EDGE_CURVE ( 'NONE', #7327, #3120, #5479, .T. ) ;
#3742=DIRECTION ( 'NONE',  ( 1.000000000000000000, 0.000000000000000000, 0.000000000000000000 ) ) ;
#3754=DIRECTION ( 'NONE',  ( 1.000000000000000000, 0.000000000000000000, 0.000000000000000000 ) ) ;
#3765=CIRCLE ( 'NONE', #5660, 8.999999999999994671 ) ;
#3773=VECTOR ( 'NONE', #7101, 1000.000000000000000 ) ;
#3799=VERTEX_POINT ( 'NONE', #3804 ) ;
#3804=CARTESIAN_POINT ( 'NONE',  ( -105.9999999999999858, -114.9999999999999858, 10.00000000000000000 ) ) ;
#3806=CARTESIAN_POINT ( 'NONE',  ( 124.0000000000000000, -114.9999999999999716, 20.00000000000000000 ) ) ;
#3817=AXIS2_PLACEMENT_3D ( 'NONE', #1903, #5006, #3742 ) ;
#3833=CARTESIAN_POINT ( 'NONE',  ( 0.000000000000000000, 0.000000000000000000, 57.99999999999999289 ) ) ;
#3851=EDGE_CURVE ( 'NONE', #653, #372, #3099, .T. ) ;
#3857=VECTOR ( 'NONE', #4468, 1000.000000000000000 ) ;
#3861=DIRECTION ( 'NONE',  ( -0.000000000000000000, -0.000000000000000000, -1.000000000000000000 ) ) ;
#3864=VERTEX_POINT ( 'NONE', #2509 ) ;
#3880=CIRCLE ( 'NONE', #1727, 5.499999999999991118 ) ;
#3892=VECTOR ( 'NONE', #5732, 1000.000000000000000 ) ;
#3901=CARTESIAN_POINT ( 'NONE',  ( 0.000000000000000000, 0.000000000000000000, 57.99999999999999289 ) ) ;
#3907=CARTESIAN_POINT ( 'NONE',  ( -124.0000000000000000, -114.9999999999999858, 20.00000000000000000 ) ) ;
#3912=EDGE_LOOP ( 'NONE', ( #1444, #2353, #4457, #6555 ) ) ;
#3913=DIRECTION ( 'NONE',  ( 0.000000000000000000, -0.000000000000000000, -1.000000000000000000 ) ) ;
#3944=( NAMED_UNIT ( * ) SI_UNIT ( $, .STERADIAN. ) SOLID_ANGLE_UNIT ( ) );
#3946=ORIENTED_EDGE ( 'NONE', *, *, #2757, .T. ) ;
#3947=DIRECTION ( 'NONE',  ( -9.992007221626408864E-16, -1.000000000000000000, 0.000000000000000000 ) ) ;
#3956=AXIS2_PLACEMENT_3D ( 'NONE', #1158, #2997, #1202 ) ;
#3964=EDGE_LOOP ( 'NONE', ( #2333, #1762, #6916, #4576 ) ) ;
#3966=FACE_BOUND ( 'NONE', #1349, .T. ) ;
#3970=FACE_OUTER_BOUND ( 'NONE', #4590, .T. ) ;
#3973=DIRECTION ( 'NONE',  ( 1.000000000000000000, 0.000000000000000000, 0.000000000000000000 ) ) ;
#3984=CYLINDRICAL_SURFACE ( 'NONE', #6042, 8.999999999999994671 ) ;
#4008=FACE_BOUND ( 'NONE', #2211, .T. ) ;
#4010=ORIENTED_EDGE ( 'NONE', *, *, #2822, .T. ) ;
#4011=DIRECTION ( 'NONE',  ( -0.000000000000000000, -0.000000000000000000, 1.000000000000000000 ) ) ;
#4018=FACE_BOUND ( 'NONE', #6888, .T. ) ;
#4022=LINE ( 'NONE', #2842, #719 ) ;
#4024=EDGE_CURVE ( 'NONE', #6262, #2853, #8040, .T. ) ;
#4027=CIRCLE ( 'NONE', #4428, 8.999999999999994671 ) ;
#4036=ORIENTED_EDGE ( 'NONE', *, *, #2588, .T. ) ;
#4052=ORIENTED_EDGE ( 'NONE', *, *, #1533, .T. ) ;
#4060=CYLINDRICAL_SURFACE ( 'NONE', #3316, 9.000000000000007105 ) ;
#4061=VECTOR ( 'NONE', #2800, 1000.000000000000000 ) ;
#4066=CIRCLE ( 'NONE', #8273, 9.000000000000007105 ) ;
#4067=CARTESIAN_POINT ( 'NONE',  ( 14.14213562373095279, -5.000000000000000000, 57.99999999999999289 ) ) ;
#4080=DIRECTION ( 'NONE',  ( -1.000000000000000000, 0.000000000000000000, -0.000000000000000000 ) ) ;
#4094=FACE_OUTER_BOUND ( 'NONE', #571, .T. ) ;
#4101=CARTESIAN_POINT ( 'NONE',  ( -109.4999999999999858, 114.9999999999999858, 0.000000000000000000 ) ) ;
#4102=ORIENTED_EDGE ( 'NONE', *, *, #2788, .T. ) ;
#4105=CARTESIAN_POINT ( 'NONE',  ( -114.9999999999999858, -114.9999999999999858, 0.000000000000000000 ) ) ;
#4107=AXIS2_PLACEMENT_3D ( 'NONE', #2522, #1898, #5172 ) ;
#4123=CARTESIAN_POINT ( 'NONE',  ( -114.9999999999999716, 114.9999999999999858, 0.000000000000000000 ) ) ;
#4142=AXIS2_PLACEMENT_3D ( 'NONE', #2288, #7432, #449 ) ;
#4146=CARTESIAN_POINT ( 'NONE',  ( -114.9999999999999858, -114.9999999999999858, 20.00000000000000000 ) ) ;
#4157=CARTESIAN_POINT ( 'NONE',  ( 115.0000000000000000, -114.9999999999999716, 20.00000000000000000 ) ) ;
#4166=DIRECTION ( 'NONE',  ( 9.992007221626408864E-16, 1.000000000000000000, 0.000000000000000000 ) ) ;
#4201=ADVANCED_FACE ( 'NONE', ( #6515, #2025 ), #4568, .T. ) ;
#4202=FACE_OUTER_BOUND ( 'NONE', #2954, .T. ) ;
#4225=FACE_OUTER_BOUND ( 'NONE', #4608, .T. ) ;
#4234=ORIENTED_EDGE ( 'NONE', *, *, #5263, .F. ) ;
#4237=ADVANCED_FACE ( 'NONE', ( #2641 ), #655, .T. ) ;
#4240=CARTESIAN_POINT ( 'NONE',  ( -120.4999999999999716, 114.9999999999999858, 10.00000000000000000 ) ) ;
#4242=CARTESIAN_POINT ( 'NONE',  ( 115.0000000000000000, 114.9999999999999716, 20.00000000000000000 ) ) ;
#4248=VECTOR ( 'NONE', #7064, 1000.000000000000000 ) ;
#4253=VECTOR ( 'NONE', #4778, 1000.000000000000000 ) ;
#4259=ORIENTED_EDGE ( 'NONE', *, *, #5406, .F. ) ;
#4264=AXIS2_PLACEMENT_3D ( 'NONE', #4157, #2852, #7386 ) ;
#4271=CARTESIAN_POINT ( 'NONE',  ( 106.0000000000000142, 114.9999999999999716, 10.00000000000000000 ) ) ;
#4282=LINE ( 'NONE', #6880, #7706 ) ;
#4285=ORIENTED_EDGE ( 'NONE', *, *, #5406, .T. ) ;
#4287=AXIS2_PLACEMENT_3D ( 'NONE', #4943, #2514, #6297 ) ;
#4296=EDGE_CURVE ( 'NONE', #5826, #3864, #4696, .T. ) ;
#4307=ORIENTED_EDGE ( 'NONE', *, *, #3223, .F. ) ;
#4350=DIRECTION ( 'NONE',  ( -0.000000000000000000, -0.000000000000000000, 1.000000000000000000 ) ) ;
#4359=UNCERTAINTY_MEASURE_WITH_UNIT (LENGTH_MEASURE( 1.000000000000000082E-05 ), #3691, 'distance_accuracy_value', 'NONE');
#4367=CYLINDRICAL_SURFACE ( 'NONE', #627, 8.999999999999994671 ) ;
#4403=CIRCLE ( 'NONE', #2545, 5.499999999999991118 ) ;
#4428=AXIS2_PLACEMENT_3D ( 'NONE', #4242, #6842, #3617 ) ;
#4433=ADVANCED_FACE ( 'NONE', ( #8162 ), #2957, .F. ) ;
#4451=FACE_OUTER_BOUND ( 'NONE', #1754, .T. ) ;
#4457=ORIENTED_EDGE ( 'NONE', *, *, #5281, .T. ) ;
#4458=ADVANCED_FACE ( 'NONE', ( #3534 ), #2909, .F. ) ;
#4468=DIRECTION ( 'NONE',  ( -0.000000000000000000, -0.000000000000000000, 1.000000000000000000 ) ) ;
#4478=CARTESIAN_POINT ( 'NONE',  ( -120.4999999999999716, 114.9999999999999858, 0.000000000000000000 ) ) ;
#4492=DIRECTION ( 'NONE',  ( -0.000000000000000000, -0.000000000000000000, 1.000000000000000000 ) ) ;
#4505=CARTESIAN_POINT ( 'NONE',  ( 124.0000000000000000, 114.9999999999999716, 20.00000000000000000 ) ) ;
#4506=DIRECTION ( 'NONE',  ( -0.000000000000000000, -0.000000000000000000, 1.000000000000000000 ) ) ;
#4508=LINE ( 'NONE', #2744, #7287 ) ;
#4509=ORIENTED_EDGE ( 'NONE', *, *, #5929, .T. ) ;
#4515=ORIENTED_EDGE ( 'NONE', *, *, #6854, .T. ) ;
#4519=DIRECTION ( 'NONE',  ( -0.000000000000000000, -0.000000000000000000, 1.000000000000000000 ) ) ;
#4548=VECTOR ( 'NONE', #322, 1000.000000000000000 ) ;
#4551=CYLINDRICAL_SURFACE ( 'NONE', #7474, 5.499999999999991118 ) ;
#4555=DIRECTION ( 'NONE',  ( -0.000000000000000000, -0.000000000000000000, 1.000000000000000000 ) ) ;
#4568=PLANE ( 'NONE',  #3315 ) ;
#4576=ORIENTED_EDGE ( 'NONE', *, *, #3415, .T. ) ;
#4578=CARTESIAN_POINT ( 'NONE',  ( 124.9999999999997442, -125.0000000000000000, 20.00000000000000000 ) ) ;
#4583=PLANE ( 'NONE',  #6991 ) ;
#4590=EDGE_LOOP ( 'NONE', ( #7012, #1644, #3124, #6368 ) ) ;
#4596=CIRCLE ( 'NONE', #3363, 8.999999999999994671 ) ;
#4604=DIRECTION ( 'NONE',  ( -0.000000000000000000, -0.000000000000000000, 1.000000000000000000 ) ) ;
#4608=EDGE_LOOP ( 'NONE', ( #7923, #1552, #6054, #5606 ) ) ;
#4617=DIRECTION ( 'NONE',  ( -0.000000000000000000, -0.000000000000000000, -1.000000000000000000 ) ) ;
#4621=PLANE ( 'NONE',  #577 ) ;
#4631=EDGE_CURVE ( 'NONE', #3543, #4652, #5751, .T. ) ;
#4652=VERTEX_POINT ( 'NONE', #4505 ) ;
#4654=LINE ( 'NONE', #7234, #4761 ) ;
#4656=CARTESIAN_POINT ( 'NONE',  ( 124.9999999999997442, -125.0000000000000000, 20.00000000000000000 ) ) ;
#4660=CARTESIAN_POINT ( 'NONE',  ( 115.0000000000000000, -114.9999999999999716, 10.00000000000000000 ) ) ;
#4663=DIRECTION ( 'NONE',  ( 1.000000000000000000, 0.000000000000000000, 0.000000000000000000 ) ) ;
#4673=DIRECTION ( 'NONE',  ( 1.000000000000000000, 0.000000000000000000, 0.000000000000000000 ) ) ;
#4688=LINE ( 'NONE', #2225, #685 ) ;
#4692=VERTEX_POINT ( 'NONE', #7788 ) ;
#4696=LINE ( 'NONE', #5996, #7925 ) ;
#4701=PLANE ( 'NONE',  #7643 ) ;
#4729=VERTEX_POINT ( 'NONE', #2823 ) ;
#4743=DIRECTION ( 'NONE',  ( 1.000000000000000000, 0.000000000000000000, 0.000000000000000000 ) ) ;
#4748=LINE ( 'NONE', #144, #3076 ) ;
#4757=ORIENTED_EDGE ( 'NONE', *, *, #8193, .T. ) ;
#4761=VECTOR ( 'NONE', #3042, 1000.000000000000000 ) ;
#4762=FACE_OUTER_BOUND ( 'NONE', #8271, .T. ) ;
#4774=ADVANCED_FACE ( 'NONE', ( #893, #4762 ), #2780, .F. ) ;
#4778=DIRECTION ( 'NONE',  ( -0.000000000000000000, -0.000000000000000000, 1.000000000000000000 ) ) ;
#4785=EDGE_CURVE ( 'NONE', #653, #5879, #3880, .T. ) ;
#4787=AXIS2_PLACEMENT_3D ( 'NONE', #3833, #4617, #7085 ) ;
#4791=ORIENTED_EDGE ( 'NONE', *, *, #7075, .F. ) ;
#4792=CYLINDRICAL_SURFACE ( 'NONE', #4264, 5.499999999999991118 ) ;
#4804=AXIS2_PLACEMENT_3D ( 'NONE', #6939, #5675, #7452 ) ;
#4807=CIRCLE ( 'NONE', #5083, 8.999999999999994671 ) ;
#4816=DIRECTION ( 'NONE',  ( 1.000000000000000000, 0.000000000000000000, 0.000000000000000000 ) ) ;
#4818=CARTESIAN_POINT ( 'NONE',  ( 20.76917701662883076, -5.000000000000000000, 0.000000000000000000 ) ) ;
#4822=DIRECTION ( 'NONE',  ( -0.000000000000000000, -0.000000000000000000, 1.000000000000000000 ) ) ;
#4823=ORIENTED_EDGE ( 'NONE', *, *, #7229, .T. ) ;
#4861=DIRECTION ( 'NONE',  ( -9.992007221626408864E-16, -1.000000000000000000, -0.000000000000000000 ) ) ;
#4875=FACE_OUTER_BOUND ( 'NONE', #2812, .T. ) ;
#4877=DIRECTION ( 'NONE',  ( -0.000000000000000000, -0.000000000000000000, 1.000000000000000000 ) ) ;
#4880=CARTESIAN_POINT ( 'NONE',  ( -125.0000000000000000, 125.0000000000000000, 20.00000000000000000 ) ) ;
#4899=AXIS2_PLACEMENT_3D ( 'NONE', #2103, #818, #4166 ) ;
#4911=FACE_OUTER_BOUND ( 'NONE', #8148, .T. ) ;
#4943=CARTESIAN_POINT ( 'NONE',  ( -114.9999999999999858, -114.9999999999999858, 20.00000000000000000 ) ) ;
#4945=( NAMED_UNIT ( * ) SI_UNIT ( $, .STERADIAN. ) SOLID_ANGLE_UNIT ( ) );
#5002=LINE ( 'NONE', #574, #6046 ) ;
#5006=DIRECTION ( 'NONE',  ( -0.000000000000000000, -0.000000000000000000, 1.000000000000000000 ) ) ;
#5016=ORIENTED_EDGE ( 'NONE', *, *, #1817, .F. ) ;
#5033=AXIS2_PLACEMENT_3D ( 'NONE', #7353, #1447, #979 ) ;
#5052=CARTESIAN_POINT ( 'NONE',  ( 75.00000000000001421, 9.184850993605150311E-15, 57.99999999999999289 ) ) ;
#5058=EDGE_CURVE ( 'NONE', #57, #758, #6451, .T. ) ;
#5083=AXIS2_PLACEMENT_3D ( 'NONE', #4660, #5173, #5850 ) ;
#5084=CARTESIAN_POINT ( 'NONE',  ( -105.9999999999999858, -114.9999999999999858, 20.00000000000000000 ) ) ;
#5090=VERTEX_POINT ( 'NONE', #2584 ) ;
#5124=DIRECTION ( 'NONE',  ( 1.000000000000000000, 0.000000000000000000, 0.000000000000000000 ) ) ;
#5129=LINE ( 'NONE', #7729, #4253 ) ;
#5141=ORIENTED_EDGE ( 'NONE', *, *, #2429, .F. ) ;
#5144=ORIENTED_EDGE ( 'NONE', *, *, #8324, .F. ) ;
#5153=EDGE_LOOP ( 'NONE', ( #2533, #7421, #99, #6130 ) ) ;
#5155=CIRCLE ( 'NONE', #1519, 5.499999999999991118 ) ;
#5172=DIRECTION ( 'NONE',  ( 1.000000000000000000, 0.000000000000000000, 0.000000000000000000 ) ) ;
#5173=DIRECTION ( 'NONE',  ( -0.000000000000000000, -0.000000000000000000, 1.000000000000000000 ) ) ;
#5174=ORIENTED_EDGE ( 'NONE', *, *, #3345, .F. ) ;
#5177=ORIENTED_EDGE ( 'NONE', *, *, #4631, .T. ) ;
#5182=CYLINDRICAL_SURFACE ( 'NONE', #2645, 5.499999999999991118 ) ;
#5183=CIRCLE ( 'NONE', #1417, 5.499999999999991118 ) ;
#5186=VERTEX_POINT ( 'NONE', #7302 ) ;
#5189=EDGE_LOOP ( 'NONE', ( #3019, #5568 ) ) ;
#5198=DIRECTION ( 'NONE',  ( -0.000000000000000000, -0.000000000000000000, 1.000000000000000000 ) ) ;
#5201=DIRECTION ( 'NONE',  ( 0.000000000000000000, 0.000000000000000000, 1.000000000000000000 ) ) ;
#5203=DIRECTION ( 'NONE',  ( 0.000000000000000000, 0.000000000000000000, 1.000000000000000000 ) ) ;
#5206=EDGE_CURVE ( 'NONE', #5879, #653, #4403, .T. ) ;
#5215=ADVANCED_FACE ( 'NONE', ( #5316 ), #6578, .F. ) ;
#5217=EDGE_CURVE ( 'NONE', #1087, #2241, #7533, .T. ) ;
#5224=EDGE_CURVE ( 'NONE', #1294, #1087, #1477, .T. ) ;
#5232=VECTOR ( 'NONE', #1557, 1000.000000000000000 ) ;
#5238=VECTOR ( 'NONE', #5834, 1000.000000000000000 ) ;
#5244=FACE_BOUND ( 'NONE', #3060, .T. ) ;
#5263=EDGE_CURVE ( 'NONE', #1889, #7860, #3433, .T. ) ;
#5281=EDGE_CURVE ( 'NONE', #7159, #2214, #1358, .T. ) ;
#5287=DIRECTION ( 'NONE',  ( -0.000000000000000000, -0.000000000000000000, 1.000000000000000000 ) ) ;
#5294=DIRECTION ( 'NONE',  ( 1.000000000000000000, 0.000000000000000000, -0.000000000000000000 ) ) ;
#5296=ORIENTED_EDGE ( 'NONE', *, *, #7340, .F. ) ;
#5306=ADVANCED_FACE ( 'NONE', ( #3017 ), #6701, .F. ) ;
#5313=CIRCLE ( 'NONE', #5033, 8.999999999999994671 ) ;
#5314=EDGE_CURVE ( 'NONE', #2083, #758, #6872, .T. ) ;
#5316=FACE_OUTER_BOUND ( 'NONE', #2231, .T. ) ;
#5319=VECTOR ( 'NONE', #5198, 1000.000000000000000 ) ;
#5331=DIRECTION ( 'NONE',  ( 1.000000000000000000, 0.000000000000000000, 0.000000000000000000 ) ) ;
#5337=DIRECTION ( 'NONE',  ( 1.000000000000000000, 0.000000000000000000, 0.000000000000000000 ) ) ;
#5351=DIRECTION ( 'NONE',  ( 1.000000000000000000, 0.000000000000000000, 0.000000000000000000 ) ) ;
#5352=VERTEX_POINT ( 'NONE', #4271 ) ;
#5358=AXIS2_PLACEMENT_3D ( 'NONE', #5360, #5405, #4080 ) ;
#5360=CARTESIAN_POINT ( 'NONE',  ( -109.4999999999999858, 114.9999999999999858, 10.00000000000000000 ) ) ;
#5368=ADVANCED_FACE ( 'NONE', ( #971 ), #4792, .F. ) ;
#5379=DIRECTION ( 'NONE',  ( 1.000000000000000000, 0.000000000000000000, 0.000000000000000000 ) ) ;
#5386=DIRECTION ( 'NONE',  ( -0.000000000000000000, -0.000000000000000000, 1.000000000000000000 ) ) ;
#5388=ORIENTED_EDGE ( 'NONE', *, *, #3036, .T. ) ;
#5392=DIRECTION ( 'NONE',  ( 1.000000000000000000, 0.000000000000000000, 0.000000000000000000 ) ) ;
#5400=ORIENTED_EDGE ( 'NONE', *, *, #3036, .F. ) ;
#5403=ADVANCED_FACE ( 'NONE', ( #2890, #8050 ), #5481, .F. ) ;
#5405=DIRECTION ( 'NONE',  ( 0.000000000000000000, 0.000000000000000000, -1.000000000000000000 ) ) ;
#5406=EDGE_CURVE ( 'NONE', #268, #5618, #1200, .T. ) ;
#5409=CARTESIAN_POINT ( 'NONE',  ( 124.9999999999997442, -125.0000000000000000, 0.000000000000000000 ) ) ;
#5411=CARTESIAN_POINT ( 'NONE',  ( -0.000000000000000000, 5.000000000000000000, 57.99999999999999289 ) ) ;
#5412=ORIENTED_EDGE ( 'NONE', *, *, #2228, .T. ) ;
#5449=CARTESIAN_POINT ( 'NONE',  ( -105.9999999999999858, 114.9999999999999858, 20.00000000000000000 ) ) ;
#5466=EDGE_LOOP ( 'NONE', ( #1366, #1538, #4307, #8192 ) ) ;
#5468=VECTOR ( 'NONE', #5379, 1000.000000000000000 ) ;
#5471=DIRECTION ( 'NONE',  ( 1.000000000000000000, 0.000000000000000000, 0.000000000000000000 ) ) ;
#5479=CIRCLE ( 'NONE', #1848, 15.00000000000000178 ) ;
#5481=PLANE ( 'NONE',  #4142 ) ;
#5493=AXIS2_PLACEMENT_3D ( 'NONE', #7326, #3457, #2274 ) ;
#5498=VECTOR ( 'NONE', #8333, 1000.000000000000000 ) ;
#5499=ORIENTED_EDGE ( 'NONE', *, *, #5930, .F. ) ;
#5508=VECTOR ( 'NONE', #73, 1000.000000000000000 ) ;
#5527=CARTESIAN_POINT ( 'NONE',  ( 125.0000000000000000, 125.0000000000000000, 20.00000000000000000 ) ) ;
#5550=( LENGTH_UNIT ( ) NAMED_UNIT ( * ) SI_UNIT ( .MILLI., .METRE. ) );
#5563=EDGE_CURVE ( 'NONE', #351, #3530, #586, .T. ) ;
#5568=ORIENTED_EDGE ( 'NONE', *, *, #4785, .T. ) ;
#5576=ORIENTED_EDGE ( 'NONE', *, *, #5918, .T. ) ;
#5581=DIRECTION ( 'NONE',  ( 1.000000000000000000, 0.000000000000000000, 0.000000000000000000 ) ) ;
#5594=ORIENTED_EDGE ( 'NONE', *, *, #1208, .T. ) ;
#5606=ORIENTED_EDGE ( 'NONE', *, *, #1533, .F. ) ;
#5609=DIRECTION ( 'NONE',  ( 0.000000000000000000, -0.000000000000000000, -1.000000000000000000 ) ) ;
#5614=CARTESIAN_POINT ( 'NONE',  ( 124.0000000000000000, -114.9999999999999716, 10.00000000000000000 ) ) ;
#5618=VERTEX_POINT ( 'NONE', #669 ) ;
#5631=ORIENTED_EDGE ( 'NONE', *, *, #2056, .F. ) ;
#5638=ADVANCED_FACE ( 'NONE', ( #2042 ), #4583, .F. ) ;
#5640=EDGE_LOOP ( 'NONE', ( #3242, #6662, #6721, #6836 ) ) ;
#5655=CARTESIAN_POINT ( 'NONE',  ( -114.9999999999999716, 114.9999999999999858, 10.00000000000000000 ) ) ;
#5660=AXIS2_PLACEMENT_3D ( 'NONE', #6263, #6987, #6312 ) ;
#5675=DIRECTION ( 'NONE',  ( -0.000000000000000000, -0.000000000000000000, 1.000000000000000000 ) ) ;
#5686=ADVANCED_FACE ( 'NONE', ( #2082 ), #3984, .F. ) ;
#5695=DIRECTION ( 'NONE',  ( 0.000000000000000000, 0.000000000000000000, 1.000000000000000000 ) ) ;
#5703=AXIS2_PLACEMENT_3D ( 'NONE', #8120, #4011, #5331 ) ;
#5708=ORIENTED_EDGE ( 'NONE', *, *, #8258, .T. ) ;
#5718=CARTESIAN_POINT ( 'NONE',  ( -120.4999999999999716, 114.9999999999999858, 20.00000000000000000 ) ) ;
#5729=ORIENTED_EDGE ( 'NONE', *, *, #1966, .F. ) ;
#5732=DIRECTION ( 'NONE',  ( 1.000000000000000000, 0.000000000000000000, 0.000000000000000000 ) ) ;
#5740=DIRECTION ( 'NONE',  ( 1.000000000000000000, 0.000000000000000000, 0.000000000000000000 ) ) ;
#5748=LINE ( 'NONE', #7177, #3857 ) ;
#5751=LINE ( 'NONE', #1368, #5498 ) ;
#5794=ORIENTED_EDGE ( 'NONE', *, *, #8207, .F. ) ;
#5812=ORIENTED_EDGE ( 'NONE', *, *, #1189, .F. ) ;
#5826=VERTEX_POINT ( 'NONE', #8124 ) ;
#5834=DIRECTION ( 'NONE',  ( -0.000000000000000000, -0.000000000000000000, -1.000000000000000000 ) ) ;
#5844=DIRECTION ( 'NONE',  ( 1.000000000000000000, 0.000000000000000000, -0.000000000000000000 ) ) ;
#5850=DIRECTION ( 'NONE',  ( 1.000000000000000000, 0.000000000000000000, 0.000000000000000000 ) ) ;
#5875=CARTESIAN_POINT ( 'NONE',  ( 0.000000000000000000, 0.000000000000000000, 20.00000000000000000 ) ) ;
#5879=VERTEX_POINT ( 'NONE', #4101 ) ;
#5884=CARTESIAN_POINT ( 'NONE',  ( 0.000000000000000000, 0.000000000000000000, 0.000000000000000000 ) ) ;
#5891=EDGE_LOOP ( 'NONE', ( #3704, #218, #8320, #634 ) ) ;
#5892=CARTESIAN_POINT ( 'NONE',  ( 115.0000000000000000, 114.9999999999999716, 20.00000000000000000 ) ) ;
#5893=VECTOR ( 'NONE', #6122, 1000.000000000000000 ) ;
#5901=ORIENTED_EDGE ( 'NONE', *, *, #5563, .T. ) ;
#5918=EDGE_CURVE ( 'NONE', #4729, #14, #7414, .T. ) ;
#5926=LINE ( 'NONE', #133, #1750 ) ;
#5927=DIRECTION ( 'NONE',  ( 1.000000000000000000, 0.000000000000000000, 0.000000000000000000 ) ) ;
#5929=EDGE_CURVE ( 'NONE', #5186, #3530, #6904, .T. ) ;
#5930=EDGE_CURVE ( 'NONE', #7972, #2241, #732, .T. ) ;
#5932=CARTESIAN_POINT ( 'NONE',  ( 20.76917701662883076, 0.000000000000000000, 0.000000000000000000 ) ) ;
#5947=CARTESIAN_POINT ( 'NONE',  ( 120.5000000000000000, -114.9999999999999716, 10.00000000000000000 ) ) ;
#5952=PLANE ( 'NONE',  #1958 ) ;
#5975=ORIENTED_EDGE ( 'NONE', *, *, #7055, .T. ) ;
#5982=ORIENTED_EDGE ( 'NONE', *, *, #8324, .T. ) ;
#5987=CARTESIAN_POINT ( 'NONE',  ( 75.00000000000001421, 9.184850993605150311E-15, 20.00000000000000000 ) ) ;
#5992=ORIENTED_EDGE ( 'NONE', *, *, #462, .T. ) ;
#5996=CARTESIAN_POINT ( 'NONE',  ( -75.00000000000001421, 0.000000000000000000, 57.99999999999999289 ) ) ;
#6010=CARTESIAN_POINT ( 'NONE',  ( -114.9999999999999858, -114.9999999999999858, 10.00000000000000000 ) ) ;
#6015=EDGE_LOOP ( 'NONE', ( #601, #2555 ) ) ;
#6016=ORIENTED_EDGE ( 'NONE', *, *, #1089, .T. ) ;
#6017=CARTESIAN_POINT ( 'NONE',  ( -125.0000000000002558, -125.0000000000000000, 20.00000000000000000 ) ) ;
#6018=EDGE_LOOP ( 'NONE', ( #7174, #7977, #6816, #7200 ) ) ;
#6022=VECTOR ( 'NONE', #2524, 1000.000000000000000 ) ;
#6032=ORIENTED_EDGE ( 'NONE', *, *, #619, .F. ) ;
#6042=AXIS2_PLACEMENT_3D ( 'NONE', #5892, #794, #4663 ) ;
#6046=VECTOR ( 'NONE', #616, 1000.000000000000000 ) ;
#6054=ORIENTED_EDGE ( 'NONE', *, *, #2912, .T. ) ;
#6069=EDGE_CURVE ( 'NONE', #6508, #1566, #7008, .T. ) ;
#6099=ORIENTED_EDGE ( 'NONE', *, *, #8128, .T. ) ;
#6122=DIRECTION ( 'NONE',  ( -0.000000000000000000, -0.000000000000000000, 1.000000000000000000 ) ) ;
#6130=ORIENTED_EDGE ( 'NONE', *, *, #284, .F. ) ;
#6154=DIRECTION ( 'NONE',  ( 1.000000000000000000, 0.000000000000000000, 0.000000000000000000 ) ) ;
#6162=AXIS2_PLACEMENT_3D ( 'NONE', #1740, #22, #7570 ) ;
#6176=CARTESIAN_POINT ( 'NONE',  ( 109.5000000000000142, -114.9999999999999716, 10.00000000000000000 ) ) ;
#6191=DIRECTION ( 'NONE',  ( 1.000000000000000000, 0.000000000000000000, 0.000000000000000000 ) ) ;
#6208=ORIENTED_EDGE ( 'NONE', *, *, #4024, .F. ) ;
#6209=CIRCLE ( 'NONE', #6, 75.00000000000001421 ) ;
#6210=CARTESIAN_POINT ( 'NONE',  ( -125.0000000000002558, -125.0000000000000000, 20.00000000000000000 ) ) ;
#6228=ADVANCED_FACE ( 'NONE', ( #4202 ), #2380, .F. ) ;
#6236=DIRECTION ( 'NONE',  ( 0.000000000000000000, -1.000000000000000000, 0.000000000000000000 ) ) ;
#6240=CARTESIAN_POINT ( 'NONE',  ( 115.0000000000000000, 114.9999999999999716, 20.00000000000000000 ) ) ;
#6262=VERTEX_POINT ( 'NONE', #3033 ) ;
#6263=CARTESIAN_POINT ( 'NONE',  ( -114.9999999999999716, 114.9999999999999858, 20.00000000000000000 ) ) ;
#6282=AXIS2_PLACEMENT_3D ( 'NONE', #6509, #5203, #5294 ) ;
#6297=DIRECTION ( 'NONE',  ( 1.000000000000000000, 0.000000000000000000, 0.000000000000000000 ) ) ;
#6301=EDGE_CURVE ( 'NONE', #293, #4652, #4027, .T. ) ;
#6304=ORIENTED_EDGE ( 'NONE', *, *, #2915, .F. ) ;
#6312=DIRECTION ( 'NONE',  ( 1.000000000000000000, 0.000000000000000000, 0.000000000000000000 ) ) ;
#6314=DIRECTION ( 'NONE',  ( 1.000000000000000000, 0.000000000000000000, 0.000000000000000000 ) ) ;
#6317=AXIS2_PLACEMENT_3D ( 'NONE', #4880, #3476, #274 ) ;
#6323=CIRCLE ( 'NONE', #2036, 5.499999999999991118 ) ;
#6338=VERTEX_POINT ( 'NONE', #8244 ) ;
#6340=EDGE_CURVE ( 'NONE', #2853, #5618, #7398, .T. ) ;
#6360=EDGE_LOOP ( 'NONE', ( #1431, #6824 ) ) ;
#6368=ORIENTED_EDGE ( 'NONE', *, *, #5224, .F. ) ;
#6396=CARTESIAN_POINT ( 'NONE',  ( 0.000000000000000000, -5.000000000000000000, 0.000000000000000000 ) ) ;
#6397=ORIENTED_EDGE ( 'NONE', *, *, #1744, .F. ) ;
#6399=CARTESIAN_POINT ( 'NONE',  ( 14.14213562373095279, 5.000000000000000000, 0.000000000000000000 ) ) ;
#6418=ORIENTED_EDGE ( 'NONE', *, *, #462, .F. ) ;
#6449=CARTESIAN_POINT ( 'NONE',  ( -109.5000000000000000, -114.9999999999999858, 0.000000000000000000 ) ) ;
#6451=LINE ( 'NONE', #8241, #790 ) ;
#6459=FACE_OUTER_BOUND ( 'NONE', #5466, .T. ) ;
#6475=DIRECTION ( 'NONE',  ( 1.000000000000000000, 0.000000000000000000, 0.000000000000000000 ) ) ;
#6482=ORIENTED_EDGE ( 'NONE', *, *, #4296, .T. ) ;
#6493=CARTESIAN_POINT ( 'NONE',  ( 20.76917701662883076, 0.000000000000000000, 57.99999999999999289 ) ) ;
#6499=ORIENTED_EDGE ( 'NONE', *, *, #4296, .F. ) ;
#6508=VERTEX_POINT ( 'NONE', #5947 ) ;
#6509=CARTESIAN_POINT ( 'NONE',  ( 0.000000000000000000, 0.000000000000000000, 20.00000000000000000 ) ) ;
#6515=FACE_BOUND ( 'NONE', #3912, .T. ) ;
#6516=CARTESIAN_POINT ( 'NONE',  ( 14.14213562373095279, 5.000000000000000000, 57.99999999999999289 ) ) ;
#6537=ORIENTED_EDGE ( 'NONE', *, *, #7806, .F. ) ;
#6546=LINE ( 'NONE', #771, #5238 ) ;
#6555=ORIENTED_EDGE ( 'NONE', *, *, #7578, .F. ) ;
#6559=AXIS2_PLACEMENT_3D ( 'NONE', #6740, #1131, #1673 ) ;
#6578=CYLINDRICAL_SURFACE ( 'NONE', #7258, 5.499999999999991118 ) ;
#6591=CARTESIAN_POINT ( 'NONE',  ( -114.9999999999999858, -114.9999999999999858, 20.00000000000000000 ) ) ;
#6600=FACE_BOUND ( 'NONE', #2309, .T. ) ;
#6606=PRODUCT ( 'Lid', 'Lid', '', ( #1187 ) ) ;
#6615=CARTESIAN_POINT ( 'NONE',  ( 0.000000000000000000, -5.000000000000000000, 0.000000000000000000 ) ) ;
#6632=CARTESIAN_POINT ( 'NONE',  ( 115.0000000000000000, -114.9999999999999716, 20.00000000000000000 ) ) ;
#6648=EDGE_CURVE ( 'NONE', #7972, #1294, #1065, .T. ) ;
#6649=CARTESIAN_POINT ( 'NONE',  ( -109.5000000000000000, -114.9999999999999858, 10.00000000000000000 ) ) ;
#6650=FACE_OUTER_BOUND ( 'NONE', #2361, .T. ) ;
#6659=DIRECTION ( 'NONE',  ( 1.000000000000000000, 0.000000000000000000, 0.000000000000000000 ) ) ;
#6662=ORIENTED_EDGE ( 'NONE', *, *, #5314, .F. ) ;
#6666=VECTOR ( 'NONE', #2187, 1000.000000000000000 ) ;
#6669=CARTESIAN_POINT ( 'NONE',  ( -125.0000000000000000, 125.0000000000000000, 20.00000000000000000 ) ) ;
#6682=LINE ( 'NONE', #905, #253 ) ;
#6689=EDGE_CURVE ( 'NONE', #1199, #6338, #1887, .T. ) ;
#6692=ORIENTED_EDGE ( 'NONE', *, *, #1817, .T. ) ;
#6694=DIRECTION ( 'NONE',  ( 1.000000000000000000, 0.000000000000000000, 0.000000000000000000 ) ) ;
#6699=CIRCLE ( 'NONE', #3057, 8.999999999999994671 ) ;
#6701=PLANE ( 'NONE',  #6317 ) ;
#6712=AXIS2_PLACEMENT_3D ( 'NONE', #3352, #3425, #6694 ) ;
#6715=ORIENTED_EDGE ( 'NONE', *, *, #8193, .F. ) ;
#6721=ORIENTED_EDGE ( 'NONE', *, *, #3415, .F. ) ;
#6725=DIRECTION ( 'NONE',  ( -0.000000000000000000, 0.000000000000000000, 1.000000000000000000 ) ) ;
#6740=CARTESIAN_POINT ( 'NONE',  ( 0.000000000000000000, 0.000000000000000000, 57.99999999999999289 ) ) ;
#6743=ORIENTED_EDGE ( 'NONE', *, *, #2767, .F. ) ;
#6744=FACE_OUTER_BOUND ( 'NONE', #2748, .T. ) ;
#6755=CARTESIAN_POINT ( 'NONE',  ( 106.0000000000000142, 114.9999999999999716, 20.00000000000000000 ) ) ;
#6758=DIRECTION ( 'NONE',  ( -0.000000000000000000, -0.000000000000000000, 1.000000000000000000 ) ) ;
#6762=DIRECTION ( 'NONE',  ( 0.000000000000000000, -0.000000000000000000, 1.000000000000000000 ) ) ;
#6768=CARTESIAN_POINT ( 'NONE',  ( 120.5000000000000000, 114.9999999999999716, 0.000000000000000000 ) ) ;
#6773=DIRECTION ( 'NONE',  ( -0.000000000000000000, -0.000000000000000000, 1.000000000000000000 ) ) ;
#6781=CARTESIAN_POINT ( 'NONE',  ( 115.0000000000000000, 114.9999999999999716, 10.00000000000000000 ) ) ;
#6787=CARTESIAN_POINT ( 'NONE',  ( -125.0000000000000000, 125.0000000000000000, 0.000000000000000000 ) ) ;
#6790=LINE ( 'NONE', #369, #3136 ) ;
#6796=DIRECTION ( 'NONE',  ( -0.000000000000000000, -0.000000000000000000, 1.000000000000000000 ) ) ;
#6816=ORIENTED_EDGE ( 'NONE', *, *, #5563, .F. ) ;
#6824=ORIENTED_EDGE ( 'NONE', *, *, #6648, .T. ) ;
#6826=EDGE_LOOP ( 'NONE', ( #5174, #6692, #6099, #6499 ) ) ;
#6836=ORIENTED_EDGE ( 'NONE', *, *, #688, .T. ) ;
#6842=DIRECTION ( 'NONE',  ( -0.000000000000000000, -0.000000000000000000, 1.000000000000000000 ) ) ;
#6849=AXIS2_PLACEMENT_3D ( 'NONE', #6781, #1009, #6191 ) ;
#6854=EDGE_CURVE ( 'NONE', #6338, #1199, #3604, .T. ) ;
#6862=VERTEX_POINT ( 'NONE', #5052 ) ;
#6872=LINE ( 'NONE', #5527, #4548 ) ;
#6875=CARTESIAN_POINT ( 'NONE',  ( 0.000000000000000000, 5.000000000000000000, 0.000000000000000000 ) ) ;
#6880=CARTESIAN_POINT ( 'NONE',  ( -125.0000000000002558, -125.0000000000000000, 20.00000000000000000 ) ) ;
#6884=CARTESIAN_POINT ( 'NONE',  ( 115.0000000000000000, -114.9999999999999716, 20.00000000000000000 ) ) ;
#6888=EDGE_LOOP ( 'NONE', ( #5812, #4259 ) ) ;
#6901=DIRECTION ( 'NONE',  ( 1.000000000000000000, 0.000000000000000000, 0.000000000000000000 ) ) ;
#6904=LINE ( 'NONE', #2444, #3773 ) ;
#6909=DIRECTION ( 'NONE',  ( -0.000000000000000000, -0.000000000000000000, 1.000000000000000000 ) ) ;
#6912=CARTESIAN_POINT ( 'NONE',  ( 14.14213562373095279, 5.000000000000000000, 0.000000000000000000 ) ) ;
#6913=ORIENTED_EDGE ( 'NONE', *, *, #7179, .T. ) ;
#6916=ORIENTED_EDGE ( 'NONE', *, *, #5263, .T. ) ;
#6922=DIRECTION ( 'NONE',  ( 1.000000000000000000, 0.000000000000000000, 0.000000000000000000 ) ) ;
#6939=CARTESIAN_POINT ( 'NONE',  ( 115.0000000000000000, 114.9999999999999716, 20.00000000000000000 ) ) ;
#6957=ORIENTED_EDGE ( 'NONE', *, *, #7065, .T. ) ;
#6959=CARTESIAN_POINT ( 'NONE',  ( 115.0000000000000000, -114.9999999999999716, 20.00000000000000000 ) ) ;
#6964=CARTESIAN_POINT ( 'NONE',  ( 0.000000000000000000, 0.000000000000000000, 57.99999999999999289 ) ) ;
#6985=DIRECTION ( 'NONE',  ( -1.000000000000000000, 0.000000000000000000, 0.000000000000000000 ) ) ;
#6987=DIRECTION ( 'NONE',  ( -0.000000000000000000, -0.000000000000000000, 1.000000000000000000 ) ) ;
#6991=AXIS2_PLACEMENT_3D ( 'NONE', #6615, #7293, #3913 ) ;
#7002=FACE_OUTER_BOUND ( 'NONE', #5153, .T. ) ;
#7003=ORIENTED_EDGE ( 'NONE', *, *, #6301, .F. ) ;
#7008=CIRCLE ( 'NONE', #7948, 5.499999999999991118 ) ;
#7009=EDGE_CURVE ( 'NONE', #426, #929, #4748, .T. ) ;
#7012=ORIENTED_EDGE ( 'NONE', *, *, #6648, .F. ) ;
#7031=CARTESIAN_POINT ( 'NONE',  ( -114.9999999999999716, 114.9999999999999858, 10.00000000000000000 ) ) ;
#7037=ORIENTED_EDGE ( 'NONE', *, *, #7055, .F. ) ;
#7044=CYLINDRICAL_SURFACE ( 'NONE', #4787, 75.00000000000001421 ) ;
#7055=EDGE_CURVE ( 'NONE', #1566, #6508, #107, .T. ) ;
#7060=DIRECTION ( 'NONE',  ( 1.000000000000000000, 0.000000000000000000, 0.000000000000000000 ) ) ;
#7064=DIRECTION ( 'NONE',  ( -0.000000000000000000, -0.000000000000000000, 1.000000000000000000 ) ) ;
#7065=EDGE_CURVE ( 'NONE', #14, #4729, #6323, .T. ) ;
#7075=EDGE_CURVE ( 'NONE', #426, #1143, #3085, .T. ) ;
#7078=EDGE_LOOP ( 'NONE', ( #5412, #2701 ) ) ;
#7085=DIRECTION ( 'NONE',  ( -1.000000000000000000, 0.000000000000000000, 0.000000000000000000 ) ) ;
#7088=DIRECTION ( 'NONE',  ( 9.992007221626408864E-16, 1.000000000000000000, 0.000000000000000000 ) ) ;
#7101=DIRECTION ( 'NONE',  ( 0.000000000000000000, -1.000000000000000000, 0.000000000000000000 ) ) ;
#7118=AXIS2_PLACEMENT_3D ( 'NONE', #3556, #919, #6659 ) ;
#7138=AXIS2_PLACEMENT_3D ( 'NONE', #7460, #5386, #2198 ) ;
#7150=ORIENTED_EDGE ( 'NONE', *, *, #7009, .F. ) ;
#7158=CARTESIAN_POINT ( 'NONE',  ( -114.9999999999999716, 114.9999999999999858, 20.00000000000000000 ) ) ;
#7159=VERTEX_POINT ( 'NONE', #2845 ) ;
#7167=EDGE_LOOP ( 'NONE', ( #6957, #5576 ) ) ;
#7174=ORIENTED_EDGE ( 'NONE', *, *, #7578, .T. ) ;
#7177=CARTESIAN_POINT ( 'NONE',  ( 109.5000000000000142, 114.9999999999999716, 20.00000000000000000 ) ) ;
#7179=EDGE_CURVE ( 'NONE', #153, #1207, #3765, .T. ) ;
#7183=AXIS2_PLACEMENT_3D ( 'NONE', #2325, #4877, #8181 ) ;
#7197=LINE ( 'NONE', #3339, #5468 ) ;
#7199=CYLINDRICAL_SURFACE ( 'NONE', #1721, 8.999999999999994671 ) ;
#7200=ORIENTED_EDGE ( 'NONE', *, *, #7340, .T. ) ;
#7201=CARTESIAN_POINT ( 'NONE',  ( -123.9999999999999716, 114.9999999999999858, 20.00000000000000000 ) ) ;
#7224=CYLINDRICAL_SURFACE ( 'NONE', #8340, 8.999999999999994671 ) ;
#7229=EDGE_CURVE ( 'NONE', #3799, #2674, #5002, .T. ) ;
#7234=CARTESIAN_POINT ( 'NONE',  ( -120.4999999999999858, -114.9999999999999858, 20.00000000000000000 ) ) ;
#7241=LINE ( 'NONE', #7768, #1192 ) ;
#7246=ORIENTED_EDGE ( 'NONE', *, *, #284, .T. ) ;
#7258=AXIS2_PLACEMENT_3D ( 'NONE', #7901, #886, #4673 ) ;
#7275=DIRECTION ( 'NONE',  ( 1.000000000000000000, 0.000000000000000000, 0.000000000000000000 ) ) ;
#7282=DIRECTION ( 'NONE',  ( -0.000000000000000000, -0.000000000000000000, -1.000000000000000000 ) ) ;
#7283=FACE_BOUND ( 'NONE', #312, .T. ) ;
#7286=DIRECTION ( 'NONE',  ( 0.000000000000000000, 0.000000000000000000, -1.000000000000000000 ) ) ;
#7287=VECTOR ( 'NONE', #4604, 1000.000000000000000 ) ;
#7293=DIRECTION ( 'NONE',  ( 0.000000000000000000, -1.000000000000000000, 0.000000000000000000 ) ) ;
#7299=DIRECTION ( 'NONE',  ( -0.000000000000000000, -0.000000000000000000, 1.000000000000000000 ) ) ;
#7302=CARTESIAN_POINT ( 'NONE',  ( 20.76917701662883076, 5.000000000000000000, 0.000000000000000000 ) ) ;
#7305=LINE ( 'NONE', #6669, #5508 ) ;
#7313=DIRECTION ( 'NONE',  ( -0.000000000000000000, 0.000000000000000000, 1.000000000000000000 ) ) ;
#7326=CARTESIAN_POINT ( 'NONE',  ( -114.9999999999999858, -114.9999999999999858, 0.000000000000000000 ) ) ;
#7327=VERTEX_POINT ( 'NONE', #6516 ) ;
#7334=CARTESIAN_POINT ( 'NONE',  ( -125.0000000000002558, -125.0000000000000000, 0.000000000000000000 ) ) ;
#7340=EDGE_CURVE ( 'NONE', #351, #3120, #5926, .T. ) ;
#7344=ORIENTED_EDGE ( 'NONE', *, *, #2429, .T. ) ;
#7349=CARTESIAN_POINT ( 'NONE',  ( -123.9999999999999716, 114.9999999999999858, 20.00000000000000000 ) ) ;
#7353=CARTESIAN_POINT ( 'NONE',  ( 115.0000000000000000, -114.9999999999999716, 20.00000000000000000 ) ) ;
#7368=DIRECTION ( 'NONE',  ( -0.000000000000000000, -0.000000000000000000, 1.000000000000000000 ) ) ;
#7378=CYLINDRICAL_SURFACE ( 'NONE', #6712, 8.999999999999994671 ) ;
#7381=CARTESIAN_POINT ( 'NONE',  ( -114.9999999999999716, 114.9999999999999858, 20.00000000000000000 ) ) ;
#7386=DIRECTION ( 'NONE',  ( 1.000000000000000000, 0.000000000000000000, 0.000000000000000000 ) ) ;
#7398=LINE ( 'NONE', #1615, #3098 ) ;
#7414=CIRCLE ( 'NONE', #7138, 5.499999999999991118 ) ;
#7415=CARTESIAN_POINT ( 'NONE',  ( -114.9999999999999716, 114.9999999999999858, 20.00000000000000000 ) ) ;
#7418=CIRCLE ( 'NONE', #119, 75.00000000000001421 ) ;
#7421=ORIENTED_EDGE ( 'NONE', *, *, #3851, .T. ) ;
#7426=CYLINDRICAL_SURFACE ( 'NONE', #873, 5.499999999999991118 ) ;
#7430=PRODUCT_DEFINITION_CONTEXT ( 'detailed design', #299, 'design' ) ;
#7432=DIRECTION ( 'NONE',  ( 0.000000000000000000, 0.000000000000000000, -1.000000000000000000 ) ) ;
#7452=DIRECTION ( 'NONE',  ( 1.000000000000000000, 0.000000000000000000, 0.000000000000000000 ) ) ;
#7460=CARTESIAN_POINT ( 'NONE',  ( 115.0000000000000000, -114.9999999999999716, 0.000000000000000000 ) ) ;
#7473=EDGE_LOOP ( 'NONE', ( #8077, #7003 ) ) ;
#7474=AXIS2_PLACEMENT_3D ( 'NONE', #6591, #5287, #768 ) ;
#7479=VERTEX_POINT ( 'NONE', #992 ) ;
#7496=CARTESIAN_POINT ( 'NONE',  ( 115.0000000000000000, 114.9999999999999716, 0.000000000000000000 ) ) ;
#7499=DIRECTION ( 'NONE',  ( -0.000000000000000000, -0.000000000000000000, 1.000000000000000000 ) ) ;
#7533=CIRCLE ( 'NONE', #3600, 8.999999999999994671 ) ;
#7537=SHAPE_REPRESENTATION_RELATIONSHIP ( 'NONE' , 'NONE' ,  #1708, #891 ) ;
#7548=CYLINDRICAL_SURFACE ( 'NONE', #8206, 5.499999999999991118 ) ;
#7559=DIRECTION ( 'NONE',  ( -0.000000000000000000, -0.000000000000000000, 1.000000000000000000 ) ) ;
#7570=DIRECTION ( 'NONE',  ( 1.000000000000000000, 0.000000000000000000, 0.000000000000000000 ) ) ;
#7571=ORIENTED_EDGE ( 'NONE', *, *, #2734, .F. ) ;
#7578=EDGE_CURVE ( 'NONE', #3120, #2214, #6682, .T. ) ;
#7627=DIRECTION ( 'NONE',  ( -0.000000000000000000, -0.000000000000000000, 1.000000000000000000 ) ) ;
#7640=AXIS2_PLACEMENT_3D ( 'NONE', #54, #3259, #6314 ) ;
#7643=AXIS2_PLACEMENT_3D ( 'NONE', #7959, #7286, #1505 ) ;
#7646=ORIENTED_EDGE ( 'NONE', *, *, #4024, .T. ) ;
#7673=CIRCLE ( 'NONE', #6162, 5.499999999999991118 ) ;
#7675=VECTOR ( 'NONE', #8013, 1000.000000000000000 ) ;
#7690=DIRECTION ( 'NONE',  ( -0.000000000000000000, -0.000000000000000000, 1.000000000000000000 ) ) ;
#7691=CARTESIAN_POINT ( 'NONE',  ( -114.9999999999999858, -114.9999999999999858, 20.00000000000000000 ) ) ;
#7694=ADVANCED_FACE ( 'NONE', ( #8294 ), #3093, .F. ) ;
#7695=ORIENTED_EDGE ( 'NONE', *, *, #8128, .F. ) ;
#7706=VECTOR ( 'NONE', #1014, 1000.000000000000000 ) ;
#7729=CARTESIAN_POINT ( 'NONE',  ( 109.5000000000000142, -114.9999999999999716, 20.00000000000000000 ) ) ;
#7738=DIRECTION ( 'NONE',  ( 1.000000000000000000, 0.000000000000000000, 0.000000000000000000 ) ) ;
#7740=ORIENTED_EDGE ( 'NONE', *, *, #51, .F. ) ;
#7766=( NAMED_UNIT ( * ) PLANE_ANGLE_UNIT ( ) SI_UNIT ( $, .RADIAN. ) );
#7768=CARTESIAN_POINT ( 'NONE',  ( -125.0000000000000000, 125.0000000000000000, 20.00000000000000000 ) ) ;
#7788=CARTESIAN_POINT ( 'NONE',  ( -124.0000000000000000, -114.9999999999999858, 10.00000000000000000 ) ) ;
#7803=DIRECTION ( 'NONE',  ( -0.000000000000000000, -0.000000000000000000, 1.000000000000000000 ) ) ;
#7806=EDGE_CURVE ( 'NONE', #3864, #1662, #1620, .T. ) ;
#7808=FACE_OUTER_BOUND ( 'NONE', #1874, .T. ) ;
#7814=ORIENTED_EDGE ( 'NONE', *, *, #5314, .T. ) ;
#7819=VECTOR ( 'NONE', #235, 1000.000000000000000 ) ;
#7833=CARTESIAN_POINT ( 'NONE',  ( 0.000000000000000000, 0.000000000000000000, 0.000000000000000000 ) ) ;
#7860=VERTEX_POINT ( 'NONE', #166 ) ;
#7862=CARTESIAN_POINT ( 'NONE',  ( 124.0000000000000000, -114.9999999999999716, 20.00000000000000000 ) ) ;
#7868=LINE ( 'NONE', #2631, #5319 ) ;
#7886=EDGE_CURVE ( 'NONE', #5186, #7159, #4508, .T. ) ;
#7901=CARTESIAN_POINT ( 'NONE',  ( 115.0000000000000000, 114.9999999999999716, 20.00000000000000000 ) ) ;
#7907=DIRECTION ( 'NONE',  ( 1.000000000000000000, 0.000000000000000000, 0.000000000000000000 ) ) ;
#7923=ORIENTED_EDGE ( 'NONE', *, *, #6854, .F. ) ;
#7925=VECTOR ( 'NONE', #7282, 1000.000000000000000 ) ;
#7941=DIRECTION ( 'NONE',  ( -0.000000000000000000, -0.000000000000000000, 1.000000000000000000 ) ) ;
#7943=PLANE ( 'NONE',  #4899 ) ;
#7946=EDGE_CURVE ( 'NONE', #758, #2041, #4688, .T. ) ;
#7948=AXIS2_PLACEMENT_3D ( 'NONE', #853, #121, #3401 ) ;
#7959=CARTESIAN_POINT ( 'NONE',  ( 120.5000000000000000, 114.9999999999999716, 10.00000000000000000 ) ) ;
#7960=AXIS2_PLACEMENT_3D ( 'NONE', #5875, #5201, #7275 ) ;
#7972=VERTEX_POINT ( 'NONE', #8236 ) ;
#7977=ORIENTED_EDGE ( 'NONE', *, *, #1698, .F. ) ;
#7980=EDGE_CURVE ( 'NONE', #7327, #7159, #898, .T. ) ;
#7985=DIRECTION ( 'NONE',  ( 1.000000000000000000, 0.000000000000000000, 0.000000000000000000 ) ) ;
#8002=DIRECTION ( 'NONE',  ( -0.000000000000000000, -0.000000000000000000, 1.000000000000000000 ) ) ;
#8006=DIRECTION ( 'NONE',  ( -0.000000000000000000, -0.000000000000000000, 1.000000000000000000 ) ) ;
#8013=DIRECTION ( 'NONE',  ( 0.000000000000000000, -1.000000000000000000, 0.000000000000000000 ) ) ;
#8014=ORIENTED_EDGE ( 'NONE', *, *, #5224, .T. ) ;
#8025=VERTEX_POINT ( 'NONE', #1053 ) ;
#8040=CIRCLE ( 'NONE', #2007, 5.499999999999991118 ) ;
#8050=FACE_OUTER_BOUND ( 'NONE', #6360, .T. ) ;
#8074=VECTOR ( 'NONE', #4350, 1000.000000000000000 ) ;
#8077=ORIENTED_EDGE ( 'NONE', *, *, #2174, .F. ) ;
#8082=ADVANCED_FACE ( 'NONE', ( #3021 ), #8139, .T. ) ;
#8086=EDGE_LOOP ( 'NONE', ( #1385, #7037 ) ) ;
#8096=CYLINDRICAL_SURFACE ( 'NONE', #7183, 15.00000000000000178 ) ;
#8103=ORIENTED_EDGE ( 'NONE', *, *, #1636, .T. ) ;
#8120=CARTESIAN_POINT ( 'NONE',  ( 115.0000000000000000, 114.9999999999999716, 10.00000000000000000 ) ) ;
#8124=CARTESIAN_POINT ( 'NONE',  ( -75.00000000000001421, 0.000000000000000000, 57.99999999999999289 ) ) ;
#8128=EDGE_CURVE ( 'NONE', #1662, #3864, #7418, .T. ) ;
#8132=CIRCLE ( 'NONE', #3956, 5.499999999999991118 ) ;
#8139=PLANE ( 'NONE',  #3625 ) ;
#8144=ADVANCED_FACE ( 'NONE', ( #7002 ), #5182, .F. ) ;
#8148=EDGE_LOOP ( 'NONE', ( #6304, #5992, #7344, #7150 ) ) ;
#8154=LINE ( 'NONE', #3411, #6666 ) ;
#8162=FACE_OUTER_BOUND ( 'NONE', #837, .T. ) ;
#8167=ADVANCED_FACE ( 'NONE', ( #2618 ), #4367, .F. ) ;
#8170=ORIENTED_EDGE ( 'NONE', *, *, #6689, .F. ) ;
#8178=AXIS2_PLACEMENT_3D ( 'NONE', #7691, #4492, #1909 ) ;
#8181=DIRECTION ( 'NONE',  ( 1.000000000000000000, 0.000000000000000000, 0.000000000000000000 ) ) ;
#8192=ORIENTED_EDGE ( 'NONE', *, *, #3525, .F. ) ;
#8193=EDGE_CURVE ( 'NONE', #2674, #7479, #3564, .T. ) ;
#8202=ADVANCED_FACE ( 'NONE', ( #4451 ), #7044, .T. ) ;
#8203=ORIENTED_EDGE ( 'NONE', *, *, #5918, .F. ) ;
#8205=VERTEX_POINT ( 'NONE', #6399 ) ;
#8206=AXIS2_PLACEMENT_3D ( 'NONE', #4146, #6909, #353 ) ;
#8207=EDGE_CURVE ( 'NONE', #5352, #3543, #482, .T. ) ;
#8236=CARTESIAN_POINT ( 'NONE',  ( 106.0000000000000142, -114.9999999999999716, 10.00000000000000000 ) ) ;
#8238=DIRECTION ( 'NONE',  ( -0.000000000000000000, -0.000000000000000000, 1.000000000000000000 ) ) ;
#8241=CARTESIAN_POINT ( 'NONE',  ( 124.9999999999997442, -125.0000000000000000, 0.000000000000000000 ) ) ;
#8244=CARTESIAN_POINT ( 'NONE',  ( -123.9999999999999716, 114.9999999999999858, 10.00000000000000000 ) ) ;
#8250=EDGE_LOOP ( 'NONE', ( #3701, #2054, #5729, #7814 ) ) ;
#8258=EDGE_CURVE ( 'NONE', #1889, #5090, #1172, .T. ) ;
#8263=CARTESIAN_POINT ( 'NONE',  ( 106.0000000000000142, -114.9999999999999716, 20.00000000000000000 ) ) ;
#8271=EDGE_LOOP ( 'NONE', ( #3392, #4515 ) ) ;
#8273=AXIS2_PLACEMENT_3D ( 'NONE', #1296, #4506, #7060 ) ;
#8285=ORIENTED_EDGE ( 'NONE', *, *, #1636, .F. ) ;
#8292=EDGE_LOOP ( 'NONE', ( #514, #924 ) ) ;
#8294=FACE_OUTER_BOUND ( 'NONE', #1165, .T. ) ;
#8298=ORIENTED_EDGE ( 'NONE', *, *, #2528, .F. ) ;
#8320=ORIENTED_EDGE ( 'NONE', *, *, #3477, .T. ) ;
#8324=EDGE_CURVE ( 'NONE', #7479, #2674, #1703, .T. ) ;
#8327=ORIENTED_EDGE ( 'NONE', *, *, #6301, .T. ) ;
#8333=DIRECTION ( 'NONE',  ( -0.000000000000000000, -0.000000000000000000, 1.000000000000000000 ) ) ;
#8340=AXIS2_PLACEMENT_3D ( 'NONE', #6632, #4555, #7985 ) ;
#8342=DIRECTION ( 'NONE',  ( 0.000000000000000000, 0.000000000000000000, 1.000000000000000000 ) ) ;
#8380=COLOUR_RGB('Light Blue',0.38,0.62,0.78);
#8381=FILL_AREA_STYLE_COLOUR('',#8380);
#8382=FILL_AREA_STYLE('',(#8381));
#8383=SURFACE_STYLE_FILL_AREA(#8382);
#8384=SURFACE_SIDE_STYLE('',(#8383));
#8385=SURFACE_STYLE_USAGE(.BOTH.,#8384);
#8386=PRESENTATION_STYLE_ASSIGNMENT((#8385));
ENDSEC;
END-ISO-10303-21;
